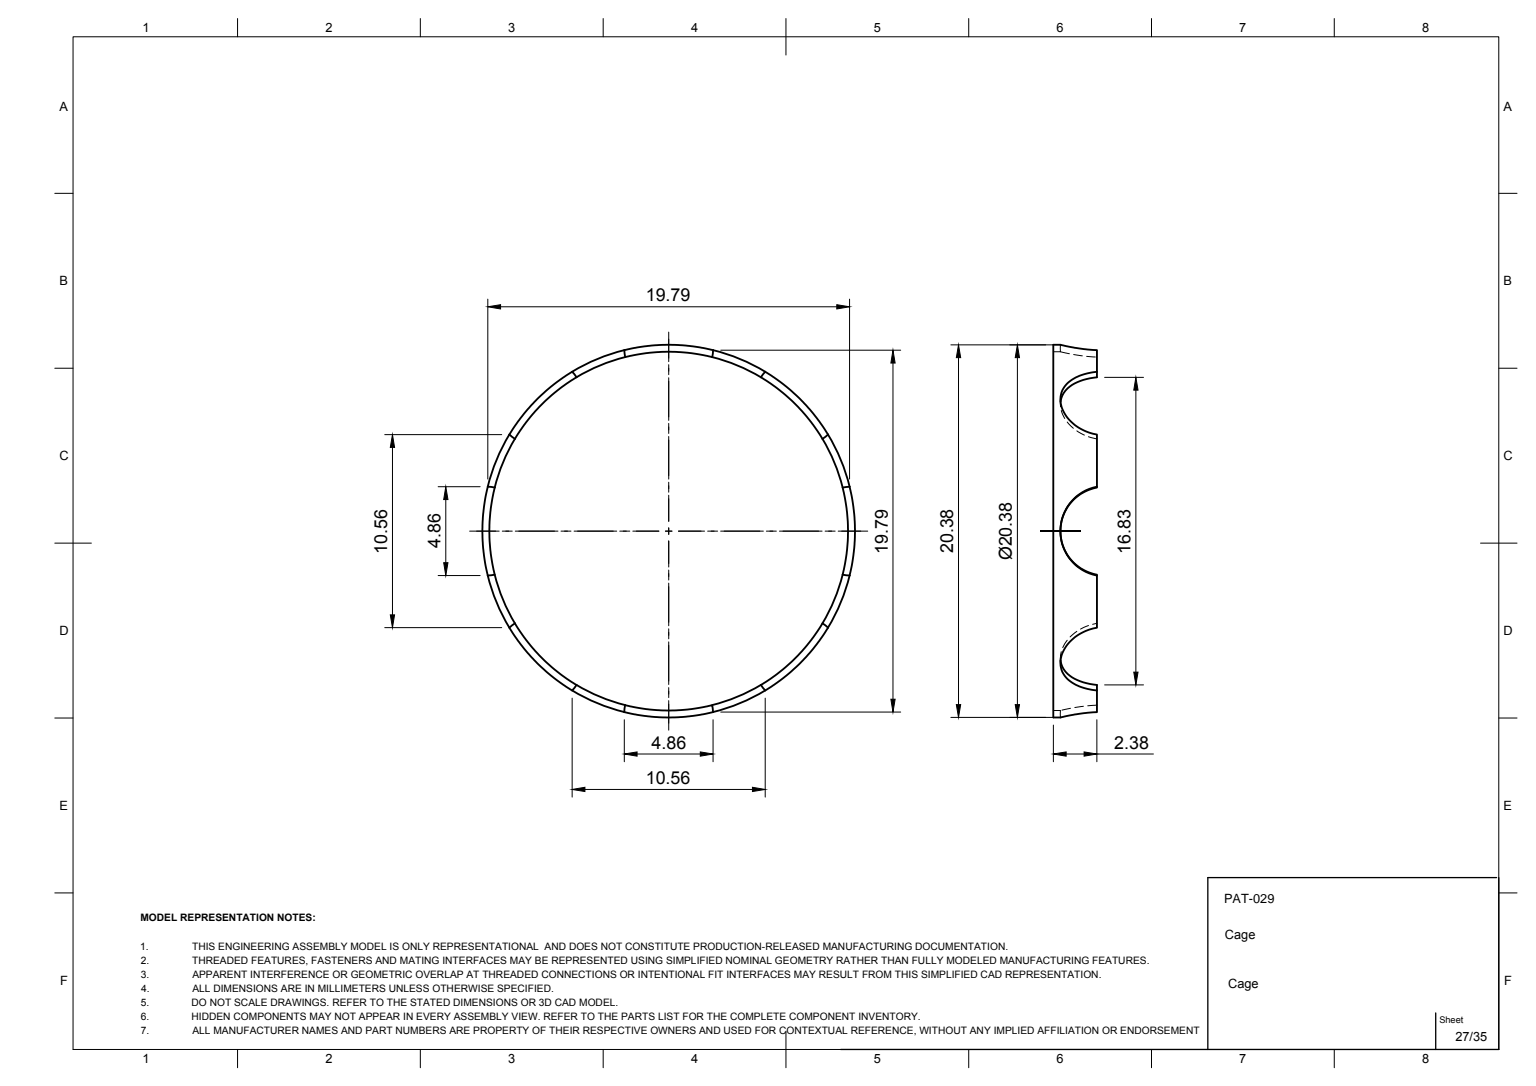
ISO-10303-21;
HEADER;
/* Generated by software containing ST-Developer
 * from STEP Tools, Inc. (www.steptools.com) 
 */

FILE_DESCRIPTION(
/* description */ ('Door-style hinge test fixture with detent'),
/* implementation_level */ '2;1');

FILE_NAME(
/* name */ 'Cage.step',
/* time_stamp */ '2026-10-28T03:24:57-07:00',
/* author */ (''),
/* organization */ (''),
/* preprocessor_version */ 'ST-DEVELOPER v20.2',
/* originating_system */ 'Autodesk Translation Framework v15.17.0.0',
/* authorisation */ '');

FILE_SCHEMA (('AUTOMOTIVE_DESIGN { 1 0 10303 214 3 1 1 }'));
ENDSEC;

DATA;
#10=MECHANICAL_DESIGN_GEOMETRIC_PRESENTATION_REPRESENTATION('',(#352),#9813);
#222=B_SPLINE_CURVE_WITH_KNOTS('',3,(#8878,#8879,#8880,#8881,#8882,#8883,
#8884,#8885,#8886,#8887,#8888,#8889,#8890,#8891,#8892,#8893,#8894,#8895,
#8896,#8897,#8898,#8899),.UNSPECIFIED.,.F.,.F.,(4,2,2,2,2,2,2,2,2,2,4),
(0.0473477652366656,0.126350602536658,0.189525903804987,0.252701205073317,
0.313298422430275,0.373895639787233,0.434492857144191,0.495090074501149,
0.558265375769478,0.621440677037807,0.7004435143378),.UNSPECIFIED.);
#223=B_SPLINE_CURVE_WITH_KNOTS('',3,(#8903,#8904,#8905,#8906,#8907,#8908,
#8909,#8910,#8911,#8912,#8913,#8914,#8915,#8916,#8917,#8918,#8919,#8920,
#8921,#8922,#8923,#8924),.UNSPECIFIED.,.F.,.F.,(4,2,2,2,2,2,2,2,2,2,4),
(0.0464897534940957,0.0852567806515119,0.170513561303024,0.246687263103517,
0.308657850341199,0.370628437578881,0.432599024816563,0.494569612054245,
0.570743313854739,0.656000094506251,0.694767121663666),.UNSPECIFIED.);
#224=B_SPLINE_CURVE_WITH_KNOTS('',3,(#8930,#8931,#8932,#8933,#8934,#8935,
#8936,#8937,#8938,#8939,#8940,#8941,#8942,#8943,#8944,#8945,#8946,#8947,
#8948,#8949,#8950,#8951),.UNSPECIFIED.,.F.,.F.,(4,2,2,2,2,2,2,2,2,2,4),
(0.0464897534940957,0.0852567806515118,0.170513561303024,0.246687263103517,
0.308657850341199,0.370628437578881,0.432599024816563,0.494569612054245,
0.570743313854738,0.65600009450625,0.694767121663666),.UNSPECIFIED.);
#225=B_SPLINE_CURVE_WITH_KNOTS('',3,(#8955,#8956,#8957,#8958,#8959,#8960,
#8961,#8962,#8963,#8964,#8965,#8966,#8967,#8968,#8969,#8970,#8971,#8972,
#8973,#8974,#8975,#8976),.UNSPECIFIED.,.F.,.F.,(4,2,2,2,2,2,2,2,2,2,4),
(0.0464897534940957,0.0852567806515119,0.170513561303024,0.246687263103517,
0.308657850341199,0.370628437578881,0.432599024816563,0.494569612054245,
0.570743313854739,0.656000094506251,0.694767121663666),.UNSPECIFIED.);
#226=B_SPLINE_CURVE_WITH_KNOTS('',3,(#8980,#8981,#8982,#8983,#8984,#8985,
#8986,#8987,#8988,#8989,#8990,#8991),.UNSPECIFIED.,.F.,.F.,(4,2,2,2,2,4),
(0.0464897534940957,0.0852567806515119,0.170513561303024,0.246687263103517,
0.308657850341199,0.370628437578881),.UNSPECIFIED.);
#227=B_SPLINE_CURVE_WITH_KNOTS('',3,(#8996,#8997,#8998,#8999,#9000,#9001,
#9002,#9003,#9004,#9005,#9006,#9007),.UNSPECIFIED.,.F.,.F.,(4,2,2,2,2,4),
(0.370628437578881,0.432599024816563,0.494569612054245,0.570743313854738,
0.65600009450625,0.694767121663666),.UNSPECIFIED.);
#228=B_SPLINE_CURVE_WITH_KNOTS('',3,(#9011,#9012,#9013,#9014,#9015,#9016,
#9017,#9018,#9019,#9020,#9021,#9022,#9023,#9024,#9025,#9026,#9027,#9028,
#9029,#9030,#9031,#9032),.UNSPECIFIED.,.F.,.F.,(4,2,2,2,2,2,2,2,2,2,4),
(0.0464897534940957,0.0852567806515121,0.170513561303024,0.246687263103518,
0.308657850341199,0.370628437578881,0.432599024816563,0.494569612054245,
0.570743313854738,0.65600009450625,0.694767121663666),.UNSPECIFIED.);
#229=B_SPLINE_CURVE_WITH_KNOTS('',3,(#9036,#9037,#9038,#9039,#9040,#9041,
#9042,#9043,#9044,#9045,#9046,#9047,#9048,#9049,#9050,#9051,#9052,#9053,
#9054,#9055,#9056,#9057),.UNSPECIFIED.,.F.,.F.,(4,2,2,2,2,2,2,2,2,2,4),
(0.0464897534940957,0.0852567806515119,0.170513561303024,0.246687263103517,
0.308657850341199,0.370628437578881,0.432599024816563,0.494569612054245,
0.570743313854738,0.65600009450625,0.694767121663667),.UNSPECIFIED.);
#230=B_SPLINE_CURVE_WITH_KNOTS('',3,(#9061,#9062,#9063,#9064,#9065,#9066,
#9067,#9068,#9069,#9070,#9071,#9072,#9073,#9074,#9075,#9076,#9077,#9078,
#9079,#9080,#9081,#9082),.UNSPECIFIED.,.F.,.F.,(4,2,2,2,2,2,2,2,2,2,4),
(0.0464897534940957,0.0852567806515119,0.170513561303024,0.246687263103517,
0.308657850341199,0.370628437578881,0.432599024816563,0.494569612054245,
0.570743313854738,0.65600009450625,0.694767121663666),.UNSPECIFIED.);
#231=B_SPLINE_CURVE_WITH_KNOTS('',3,(#9086,#9087,#9088,#9089,#9090,#9091,
#9092,#9093,#9094,#9095,#9096,#9097,#9098,#9099,#9100,#9101,#9102,#9103,
#9104,#9105,#9106,#9107),.UNSPECIFIED.,.F.,.F.,(4,2,2,2,2,2,2,2,2,2,4),
(0.0464897534940957,0.0852567806515119,0.170513561303024,0.246687263103517,
0.308657850341199,0.370628437578881,0.432599024816563,0.494569612054245,
0.570743313854739,0.656000094506251,0.694767121663667),.UNSPECIFIED.);
#232=B_SPLINE_CURVE_WITH_KNOTS('',3,(#9115,#9116,#9117,#9118,#9119,#9120,
#9121,#9122,#9123,#9124,#9125,#9126,#9127,#9128,#9129,#9130,#9131,#9132,
#9133,#9134,#9135,#9136),.UNSPECIFIED.,.F.,.F.,(4,2,2,2,2,2,2,2,2,2,4),
(0.0473477652366656,0.126350602536658,0.189525903804987,0.252701205073316,
0.313298422430274,0.373895639787232,0.434492857144191,0.495090074501149,
0.558265375769478,0.621440677037807,0.7004435143378),.UNSPECIFIED.);
#233=B_SPLINE_CURVE_WITH_KNOTS('',3,(#9144,#9145,#9146,#9147,#9148,#9149,
#9150,#9151,#9152,#9153,#9154,#9155,#9156,#9157,#9158,#9159,#9160,#9161,
#9162,#9163,#9164,#9165),.UNSPECIFIED.,.F.,.F.,(4,2,2,2,2,2,2,2,2,2,4),
(0.0473477652366656,0.126350602536658,0.189525903804987,0.252701205073317,
0.313298422430275,0.373895639787233,0.434492857144191,0.495090074501149,
0.558265375769478,0.621440677037807,0.7004435143378),.UNSPECIFIED.);
#234=B_SPLINE_CURVE_WITH_KNOTS('',3,(#9174,#9175,#9176,#9177,#9178,#9179,
#9180,#9181,#9182,#9183,#9184,#9185),.UNSPECIFIED.,.F.,.F.,(4,2,2,2,2,4),
(0.0473477652366656,0.126350602536658,0.189525903804987,0.252701205073316,
0.313298422430275,0.373895639787233),.UNSPECIFIED.);
#235=B_SPLINE_CURVE_WITH_KNOTS('',3,(#9187,#9188,#9189,#9190,#9191,#9192,
#9193,#9194,#9195,#9196,#9197,#9198),.UNSPECIFIED.,.F.,.F.,(4,2,2,2,2,4),
(0.373895639787233,0.434492857144191,0.495090074501149,0.558265375769478,
0.621440677037807,0.7004435143378),.UNSPECIFIED.);
#236=B_SPLINE_CURVE_WITH_KNOTS('',3,(#9205,#9206,#9207,#9208,#9209,#9210,
#9211,#9212,#9213,#9214,#9215,#9216,#9217,#9218,#9219,#9220,#9221,#9222,
#9223,#9224,#9225,#9226),.UNSPECIFIED.,.F.,.F.,(4,2,2,2,2,2,2,2,2,2,4),
(0.0473477652366656,0.126350602536658,0.189525903804987,0.252701205073316,
0.313298422430275,0.373895639787233,0.434492857144191,0.495090074501149,
0.558265375769478,0.621440677037807,0.7004435143378),.UNSPECIFIED.);
#237=B_SPLINE_CURVE_WITH_KNOTS('',3,(#9234,#9235,#9236,#9237,#9238,#9239,
#9240,#9241,#9242,#9243,#9244,#9245,#9246,#9247,#9248,#9249,#9250,#9251,
#9252,#9253,#9254,#9255),.UNSPECIFIED.,.F.,.F.,(4,2,2,2,2,2,2,2,2,2,4),
(0.0473477652366656,0.126350602536658,0.189525903804987,0.252701205073317,
0.313298422430275,0.373895639787233,0.434492857144191,0.495090074501149,
0.558265375769478,0.621440677037807,0.7004435143378),.UNSPECIFIED.);
#238=B_SPLINE_CURVE_WITH_KNOTS('',3,(#9263,#9264,#9265,#9266,#9267,#9268,
#9269,#9270,#9271,#9272,#9273,#9274,#9275,#9276,#9277,#9278,#9279,#9280,
#9281,#9282,#9283,#9284),.UNSPECIFIED.,.F.,.F.,(4,2,2,2,2,2,2,2,2,2,4),
(0.0473477652366656,0.126350602536658,0.189525903804987,0.252701205073316,
0.313298422430275,0.373895639787233,0.434492857144191,0.495090074501149,
0.558265375769478,0.621440677037807,0.7004435143378),.UNSPECIFIED.);
#239=B_SPLINE_CURVE_WITH_KNOTS('',3,(#9293,#9294,#9295,#9296,#9297,#9298,
#9299,#9300,#9301,#9302,#9303,#9304,#9305,#9306,#9307,#9308,#9309,#9310,
#9311,#9312,#9313,#9314),.UNSPECIFIED.,.F.,.F.,(4,2,2,2,2,2,2,2,2,2,4),
(0.0473477652366656,0.126350602536658,0.189525903804987,0.252701205073317,
0.313298422430275,0.373895639787233,0.434492857144191,0.495090074501149,
0.558265375769478,0.621440677037807,0.7004435143378),.UNSPECIFIED.);
#251=SPHERICAL_SURFACE('',#5501,0.247676);
#252=SPHERICAL_SURFACE('',#5517,0.247676);
#253=SPHERICAL_SURFACE('',#5522,0.247676);
#254=SPHERICAL_SURFACE('',#5527,0.247676);
#255=SPHERICAL_SURFACE('',#5532,0.247676);
#256=SPHERICAL_SURFACE('',#5537,0.247676);
#257=SPHERICAL_SURFACE('',#5542,0.247676);
#258=SPHERICAL_SURFACE('',#5550,0.247676);
#282=SHAPE_REPRESENTATION_RELATIONSHIP('SRR','None',#9960,#313);
#313=ADVANCED_BREP_SHAPE_REPRESENTATION('',(#391),#9803);
#352=STYLED_ITEM('',(#10183),#391);
#391=MANIFOLD_SOLID_BREP('Continuous crown cage',#4784);
#472=FACE_BOUND('',#1225,.T.);
#609=PLANE('',#5514);
#610=PLANE('',#5519);
#611=PLANE('',#5524);
#612=PLANE('',#5529);
#613=PLANE('',#5534);
#614=PLANE('',#5539);
#615=PLANE('',#5548);
#616=PLANE('',#5552);
#617=PLANE('',#5553);
#849=FACE_OUTER_BOUND('',#1207,.T.);
#850=FACE_OUTER_BOUND('',#1208,.T.);
#851=FACE_OUTER_BOUND('',#1209,.T.);
#852=FACE_OUTER_BOUND('',#1210,.T.);
#853=FACE_OUTER_BOUND('',#1211,.T.);
#854=FACE_OUTER_BOUND('',#1212,.T.);
#855=FACE_OUTER_BOUND('',#1213,.T.);
#856=FACE_OUTER_BOUND('',#1214,.T.);
#857=FACE_OUTER_BOUND('',#1215,.T.);
#858=FACE_OUTER_BOUND('',#1216,.T.);
#859=FACE_OUTER_BOUND('',#1217,.T.);
#860=FACE_OUTER_BOUND('',#1218,.T.);
#861=FACE_OUTER_BOUND('',#1219,.T.);
#862=FACE_OUTER_BOUND('',#1220,.T.);
#863=FACE_OUTER_BOUND('',#1221,.T.);
#864=FACE_OUTER_BOUND('',#1222,.T.);
#865=FACE_OUTER_BOUND('',#1223,.T.);
#866=FACE_OUTER_BOUND('',#1224,.T.);
#867=FACE_OUTER_BOUND('',#1226,.T.);
#1207=EDGE_LOOP('',(#3979,#3980,#3981,#3982));
#1208=EDGE_LOOP('',(#3983,#3984,#3985,#3986,#3987,#3988,#3989,#3990,#3991,
#3992,#3993,#3994,#3995,#3996,#3997,#3998,#3999,#4000,#4001,#4002));
#1209=EDGE_LOOP('',(#4003,#4004,#4005,#4006));
#1210=EDGE_LOOP('',(#4007,#4008,#4009,#4010));
#1211=EDGE_LOOP('',(#4011,#4012,#4013,#4014));
#1212=EDGE_LOOP('',(#4015,#4016,#4017,#4018));
#1213=EDGE_LOOP('',(#4019,#4020,#4021,#4022));
#1214=EDGE_LOOP('',(#4023,#4024,#4025,#4026,#4027,#4028));
#1215=EDGE_LOOP('',(#4029,#4030,#4031,#4032));
#1216=EDGE_LOOP('',(#4033,#4034,#4035,#4036));
#1217=EDGE_LOOP('',(#4037,#4038,#4039,#4040));
#1218=EDGE_LOOP('',(#4041,#4042,#4043,#4044));
#1219=EDGE_LOOP('',(#4045,#4046,#4047,#4048));
#1220=EDGE_LOOP('',(#4049,#4050,#4051,#4052));
#1221=EDGE_LOOP('',(#4053,#4054,#4055,#4056,#4057,#4058,#4059,#4060,#4061,
#4062,#4063,#4064,#4065,#4066,#4067,#4068,#4069,#4070,#4071,#4072));
#1222=EDGE_LOOP('',(#4073,#4074,#4075,#4076));
#1223=EDGE_LOOP('',(#4077,#4078,#4079,#4080));
#1224=EDGE_LOOP('',(#4081));
#1225=EDGE_LOOP('',(#4082));
#1226=EDGE_LOOP('',(#4083,#4084,#4085,#4086));
#1567=LINE('',#8993,#1887);
#1568=LINE('',#9289,#1888);
#1887=VECTOR('',#6724,1.019052);
#1888=VECTOR('',#6801,0.980948);
#2126=CIRCLE('',#5502,0.243053047864041);
#2127=CIRCLE('',#5503,0.243053047864041);
#2128=CIRCLE('',#5505,1.019052);
#2129=CIRCLE('',#5506,1.019052);
#2130=CIRCLE('',#5507,1.019052);
#2131=CIRCLE('',#5508,1.019052);
#2132=CIRCLE('',#5509,1.019052);
#2133=CIRCLE('',#5510,1.019052);
#2134=CIRCLE('',#5511,1.019052);
#2135=CIRCLE('',#5512,1.019052);
#2136=CIRCLE('',#5513,1.019052);
#2137=CIRCLE('',#5515,0.980948);
#2138=CIRCLE('',#5516,0.243053047864041);
#2139=CIRCLE('',#5518,0.243053047864041);
#2140=CIRCLE('',#5520,0.980948);
#2141=CIRCLE('',#5521,0.243053047864041);
#2142=CIRCLE('',#5523,0.243053047864041);
#2143=CIRCLE('',#5525,0.980948);
#2144=CIRCLE('',#5526,0.243053047864041);
#2145=CIRCLE('',#5528,0.243053047864041);
#2146=CIRCLE('',#5530,0.980948);
#2147=CIRCLE('',#5531,0.243053047864041);
#2148=CIRCLE('',#5533,0.243053047864041);
#2149=CIRCLE('',#5535,0.980948);
#2150=CIRCLE('',#5536,0.243053047864041);
#2151=CIRCLE('',#5538,0.243053047864041);
#2152=CIRCLE('',#5540,0.980948);
#2153=CIRCLE('',#5541,0.243053047864041);
#2154=CIRCLE('',#5543,0.243053047864041);
#2155=CIRCLE('',#5545,0.980948);
#2156=CIRCLE('',#5546,0.980948);
#2157=CIRCLE('',#5547,0.980948);
#2158=CIRCLE('',#5549,0.243053047864041);
#2159=CIRCLE('',#5551,0.243053047864041);
#2488=VERTEX_POINT('',#8876);
#2489=VERTEX_POINT('',#8877);
#2490=VERTEX_POINT('',#8900);
#2491=VERTEX_POINT('',#8902);
#2492=VERTEX_POINT('',#8927);
#2493=VERTEX_POINT('',#8929);
#2494=VERTEX_POINT('',#8952);
#2495=VERTEX_POINT('',#8954);
#2496=VERTEX_POINT('',#8977);
#2497=VERTEX_POINT('',#8979);
#2498=VERTEX_POINT('',#8992);
#2499=VERTEX_POINT('',#8995);
#2500=VERTEX_POINT('',#9008);
#2501=VERTEX_POINT('',#9010);
#2502=VERTEX_POINT('',#9033);
#2503=VERTEX_POINT('',#9035);
#2504=VERTEX_POINT('',#9058);
#2505=VERTEX_POINT('',#9060);
#2506=VERTEX_POINT('',#9083);
#2507=VERTEX_POINT('',#9085);
#2508=VERTEX_POINT('',#9110);
#2509=VERTEX_POINT('',#9114);
#2510=VERTEX_POINT('',#9139);
#2511=VERTEX_POINT('',#9143);
#2512=VERTEX_POINT('',#9168);
#2513=VERTEX_POINT('',#9172);
#2514=VERTEX_POINT('',#9173);
#2515=VERTEX_POINT('',#9200);
#2516=VERTEX_POINT('',#9204);
#2517=VERTEX_POINT('',#9229);
#2518=VERTEX_POINT('',#9233);
#2519=VERTEX_POINT('',#9258);
#2520=VERTEX_POINT('',#9262);
#2521=VERTEX_POINT('',#9287);
#2522=VERTEX_POINT('',#9290);
#2523=VERTEX_POINT('',#9292);
#3006=EDGE_CURVE('',#2488,#2489,#222,.T.);
#3007=EDGE_CURVE('',#2490,#2488,#2126,.T.);
#3008=EDGE_CURVE('',#2491,#2490,#223,.T.);
#3009=EDGE_CURVE('',#2489,#2491,#2127,.T.);
#3010=EDGE_CURVE('',#2492,#2490,#2128,.T.);
#3011=EDGE_CURVE('',#2492,#2493,#224,.T.);
#3012=EDGE_CURVE('',#2494,#2493,#2129,.T.);
#3013=EDGE_CURVE('',#2494,#2495,#225,.T.);
#3014=EDGE_CURVE('',#2496,#2495,#2130,.T.);
#3015=EDGE_CURVE('',#2496,#2497,#226,.T.);
#3016=EDGE_CURVE('',#2497,#2498,#1567,.T.);
#3017=EDGE_CURVE('',#2498,#2498,#2131,.T.);
#3018=EDGE_CURVE('',#2497,#2499,#227,.T.);
#3019=EDGE_CURVE('',#2500,#2499,#2132,.T.);
#3020=EDGE_CURVE('',#2500,#2501,#228,.T.);
#3021=EDGE_CURVE('',#2502,#2501,#2133,.T.);
#3022=EDGE_CURVE('',#2502,#2503,#229,.T.);
#3023=EDGE_CURVE('',#2504,#2503,#2134,.T.);
#3024=EDGE_CURVE('',#2504,#2505,#230,.T.);
#3025=EDGE_CURVE('',#2506,#2505,#2135,.T.);
#3026=EDGE_CURVE('',#2506,#2507,#231,.T.);
#3027=EDGE_CURVE('',#2491,#2507,#2136,.T.);
#3028=EDGE_CURVE('',#2488,#2508,#2137,.T.);
#3029=EDGE_CURVE('',#2508,#2492,#2138,.T.);
#3030=EDGE_CURVE('',#2509,#2508,#232,.T.);
#3031=EDGE_CURVE('',#2493,#2509,#2139,.T.);
#3032=EDGE_CURVE('',#2509,#2510,#2140,.T.);
#3033=EDGE_CURVE('',#2510,#2494,#2141,.T.);
#3034=EDGE_CURVE('',#2511,#2510,#233,.T.);
#3035=EDGE_CURVE('',#2495,#2511,#2142,.T.);
#3036=EDGE_CURVE('',#2511,#2512,#2143,.T.);
#3037=EDGE_CURVE('',#2512,#2496,#2144,.T.);
#3038=EDGE_CURVE('',#2513,#2514,#234,.T.);
#3039=EDGE_CURVE('',#2499,#2513,#2145,.T.);
#3040=EDGE_CURVE('',#2514,#2512,#235,.T.);
#3041=EDGE_CURVE('',#2513,#2515,#2146,.T.);
#3042=EDGE_CURVE('',#2515,#2500,#2147,.T.);
#3043=EDGE_CURVE('',#2516,#2515,#236,.T.);
#3044=EDGE_CURVE('',#2501,#2516,#2148,.T.);
#3045=EDGE_CURVE('',#2516,#2517,#2149,.T.);
#3046=EDGE_CURVE('',#2517,#2502,#2150,.T.);
#3047=EDGE_CURVE('',#2518,#2517,#237,.T.);
#3048=EDGE_CURVE('',#2503,#2518,#2151,.T.);
#3049=EDGE_CURVE('',#2518,#2519,#2152,.T.);
#3050=EDGE_CURVE('',#2519,#2504,#2153,.T.);
#3051=EDGE_CURVE('',#2520,#2519,#238,.T.);
#3052=EDGE_CURVE('',#2505,#2520,#2154,.T.);
#3053=EDGE_CURVE('',#2521,#2521,#2155,.T.);
#3054=EDGE_CURVE('',#2521,#2514,#1568,.T.);
#3055=EDGE_CURVE('',#2522,#2489,#2156,.T.);
#3056=EDGE_CURVE('',#2522,#2523,#239,.T.);
#3057=EDGE_CURVE('',#2520,#2523,#2157,.T.);
#3058=EDGE_CURVE('',#2507,#2522,#2158,.T.);
#3059=EDGE_CURVE('',#2523,#2506,#2159,.T.);
#3979=ORIENTED_EDGE('',*,*,#3006,.F.);
#3980=ORIENTED_EDGE('',*,*,#3007,.F.);
#3981=ORIENTED_EDGE('',*,*,#3008,.F.);
#3982=ORIENTED_EDGE('',*,*,#3009,.F.);
#3983=ORIENTED_EDGE('',*,*,#3008,.T.);
#3984=ORIENTED_EDGE('',*,*,#3010,.F.);
#3985=ORIENTED_EDGE('',*,*,#3011,.T.);
#3986=ORIENTED_EDGE('',*,*,#3012,.F.);
#3987=ORIENTED_EDGE('',*,*,#3013,.T.);
#3988=ORIENTED_EDGE('',*,*,#3014,.F.);
#3989=ORIENTED_EDGE('',*,*,#3015,.T.);
#3990=ORIENTED_EDGE('',*,*,#3016,.T.);
#3991=ORIENTED_EDGE('',*,*,#3017,.F.);
#3992=ORIENTED_EDGE('',*,*,#3016,.F.);
#3993=ORIENTED_EDGE('',*,*,#3018,.T.);
#3994=ORIENTED_EDGE('',*,*,#3019,.F.);
#3995=ORIENTED_EDGE('',*,*,#3020,.T.);
#3996=ORIENTED_EDGE('',*,*,#3021,.F.);
#3997=ORIENTED_EDGE('',*,*,#3022,.T.);
#3998=ORIENTED_EDGE('',*,*,#3023,.F.);
#3999=ORIENTED_EDGE('',*,*,#3024,.T.);
#4000=ORIENTED_EDGE('',*,*,#3025,.F.);
#4001=ORIENTED_EDGE('',*,*,#3026,.T.);
#4002=ORIENTED_EDGE('',*,*,#3027,.F.);
#4003=ORIENTED_EDGE('',*,*,#3007,.T.);
#4004=ORIENTED_EDGE('',*,*,#3028,.T.);
#4005=ORIENTED_EDGE('',*,*,#3029,.T.);
#4006=ORIENTED_EDGE('',*,*,#3010,.T.);
#4007=ORIENTED_EDGE('',*,*,#3030,.F.);
#4008=ORIENTED_EDGE('',*,*,#3031,.F.);
#4009=ORIENTED_EDGE('',*,*,#3011,.F.);
#4010=ORIENTED_EDGE('',*,*,#3029,.F.);
#4011=ORIENTED_EDGE('',*,*,#3031,.T.);
#4012=ORIENTED_EDGE('',*,*,#3032,.T.);
#4013=ORIENTED_EDGE('',*,*,#3033,.T.);
#4014=ORIENTED_EDGE('',*,*,#3012,.T.);
#4015=ORIENTED_EDGE('',*,*,#3034,.F.);
#4016=ORIENTED_EDGE('',*,*,#3035,.F.);
#4017=ORIENTED_EDGE('',*,*,#3013,.F.);
#4018=ORIENTED_EDGE('',*,*,#3033,.F.);
#4019=ORIENTED_EDGE('',*,*,#3035,.T.);
#4020=ORIENTED_EDGE('',*,*,#3036,.T.);
#4021=ORIENTED_EDGE('',*,*,#3037,.T.);
#4022=ORIENTED_EDGE('',*,*,#3014,.T.);
#4023=ORIENTED_EDGE('',*,*,#3038,.F.);
#4024=ORIENTED_EDGE('',*,*,#3039,.F.);
#4025=ORIENTED_EDGE('',*,*,#3018,.F.);
#4026=ORIENTED_EDGE('',*,*,#3015,.F.);
#4027=ORIENTED_EDGE('',*,*,#3037,.F.);
#4028=ORIENTED_EDGE('',*,*,#3040,.F.);
#4029=ORIENTED_EDGE('',*,*,#3039,.T.);
#4030=ORIENTED_EDGE('',*,*,#3041,.T.);
#4031=ORIENTED_EDGE('',*,*,#3042,.T.);
#4032=ORIENTED_EDGE('',*,*,#3019,.T.);
#4033=ORIENTED_EDGE('',*,*,#3043,.F.);
#4034=ORIENTED_EDGE('',*,*,#3044,.F.);
#4035=ORIENTED_EDGE('',*,*,#3020,.F.);
#4036=ORIENTED_EDGE('',*,*,#3042,.F.);
#4037=ORIENTED_EDGE('',*,*,#3044,.T.);
#4038=ORIENTED_EDGE('',*,*,#3045,.T.);
#4039=ORIENTED_EDGE('',*,*,#3046,.T.);
#4040=ORIENTED_EDGE('',*,*,#3021,.T.);
#4041=ORIENTED_EDGE('',*,*,#3047,.F.);
#4042=ORIENTED_EDGE('',*,*,#3048,.F.);
#4043=ORIENTED_EDGE('',*,*,#3022,.F.);
#4044=ORIENTED_EDGE('',*,*,#3046,.F.);
#4045=ORIENTED_EDGE('',*,*,#3048,.T.);
#4046=ORIENTED_EDGE('',*,*,#3049,.T.);
#4047=ORIENTED_EDGE('',*,*,#3050,.T.);
#4048=ORIENTED_EDGE('',*,*,#3023,.T.);
#4049=ORIENTED_EDGE('',*,*,#3024,.F.);
#4050=ORIENTED_EDGE('',*,*,#3050,.F.);
#4051=ORIENTED_EDGE('',*,*,#3051,.F.);
#4052=ORIENTED_EDGE('',*,*,#3052,.F.);
#4053=ORIENTED_EDGE('',*,*,#3053,.F.);
#4054=ORIENTED_EDGE('',*,*,#3054,.T.);
#4055=ORIENTED_EDGE('',*,*,#3040,.T.);
#4056=ORIENTED_EDGE('',*,*,#3036,.F.);
#4057=ORIENTED_EDGE('',*,*,#3034,.T.);
#4058=ORIENTED_EDGE('',*,*,#3032,.F.);
#4059=ORIENTED_EDGE('',*,*,#3030,.T.);
#4060=ORIENTED_EDGE('',*,*,#3028,.F.);
#4061=ORIENTED_EDGE('',*,*,#3006,.T.);
#4062=ORIENTED_EDGE('',*,*,#3055,.F.);
#4063=ORIENTED_EDGE('',*,*,#3056,.T.);
#4064=ORIENTED_EDGE('',*,*,#3057,.F.);
#4065=ORIENTED_EDGE('',*,*,#3051,.T.);
#4066=ORIENTED_EDGE('',*,*,#3049,.F.);
#4067=ORIENTED_EDGE('',*,*,#3047,.T.);
#4068=ORIENTED_EDGE('',*,*,#3045,.F.);
#4069=ORIENTED_EDGE('',*,*,#3043,.T.);
#4070=ORIENTED_EDGE('',*,*,#3041,.F.);
#4071=ORIENTED_EDGE('',*,*,#3038,.T.);
#4072=ORIENTED_EDGE('',*,*,#3054,.F.);
#4073=ORIENTED_EDGE('',*,*,#3009,.T.);
#4074=ORIENTED_EDGE('',*,*,#3027,.T.);
#4075=ORIENTED_EDGE('',*,*,#3058,.T.);
#4076=ORIENTED_EDGE('',*,*,#3055,.T.);
#4077=ORIENTED_EDGE('',*,*,#3026,.F.);
#4078=ORIENTED_EDGE('',*,*,#3059,.F.);
#4079=ORIENTED_EDGE('',*,*,#3056,.F.);
#4080=ORIENTED_EDGE('',*,*,#3058,.F.);
#4081=ORIENTED_EDGE('',*,*,#3017,.T.);
#4082=ORIENTED_EDGE('',*,*,#3053,.T.);
#4083=ORIENTED_EDGE('',*,*,#3052,.T.);
#4084=ORIENTED_EDGE('',*,*,#3057,.T.);
#4085=ORIENTED_EDGE('',*,*,#3059,.T.);
#4086=ORIENTED_EDGE('',*,*,#3025,.T.);
#4439=CYLINDRICAL_SURFACE('',#5504,1.019052);
#4440=CYLINDRICAL_SURFACE('',#5544,0.980948);
#4654=ADVANCED_FACE('',(#849),#251,.F.);
#4655=ADVANCED_FACE('',(#850),#4439,.T.);
#4656=ADVANCED_FACE('',(#851),#609,.T.);
#4657=ADVANCED_FACE('',(#852),#252,.F.);
#4658=ADVANCED_FACE('',(#853),#610,.T.);
#4659=ADVANCED_FACE('',(#854),#253,.F.);
#4660=ADVANCED_FACE('',(#855),#611,.T.);
#4661=ADVANCED_FACE('',(#856),#254,.F.);
#4662=ADVANCED_FACE('',(#857),#612,.T.);
#4663=ADVANCED_FACE('',(#858),#255,.F.);
#4664=ADVANCED_FACE('',(#859),#613,.T.);
#4665=ADVANCED_FACE('',(#860),#256,.F.);
#4666=ADVANCED_FACE('',(#861),#614,.T.);
#4667=ADVANCED_FACE('',(#862),#257,.F.);
#4668=ADVANCED_FACE('',(#863),#4440,.F.);
#4669=ADVANCED_FACE('',(#864),#615,.T.);
#4670=ADVANCED_FACE('',(#865),#258,.F.);
#4671=ADVANCED_FACE('',(#866,#472),#616,.T.);
#4672=ADVANCED_FACE('',(#867),#617,.T.);
#4784=CLOSED_SHELL('',(#4654,#4655,#4656,#4657,#4658,#4659,#4660,#4661,
#4662,#4663,#4664,#4665,#4666,#4667,#4668,#4669,#4670,#4671,#4672));
#5500=AXIS2_PLACEMENT_3D('',#8874,#6708,#6709);
#5501=AXIS2_PLACEMENT_3D('',#8875,#6710,#6711);
#5502=AXIS2_PLACEMENT_3D('',#8901,#6712,#6713);
#5503=AXIS2_PLACEMENT_3D('',#8925,#6714,#6715);
#5504=AXIS2_PLACEMENT_3D('',#8926,#6716,#6717);
#5505=AXIS2_PLACEMENT_3D('',#8928,#6718,#6719);
#5506=AXIS2_PLACEMENT_3D('',#8953,#6720,#6721);
#5507=AXIS2_PLACEMENT_3D('',#8978,#6722,#6723);
#5508=AXIS2_PLACEMENT_3D('',#8994,#6725,#6726);
#5509=AXIS2_PLACEMENT_3D('',#9009,#6727,#6728);
#5510=AXIS2_PLACEMENT_3D('',#9034,#6729,#6730);
#5511=AXIS2_PLACEMENT_3D('',#9059,#6731,#6732);
#5512=AXIS2_PLACEMENT_3D('',#9084,#6733,#6734);
#5513=AXIS2_PLACEMENT_3D('',#9108,#6735,#6736);
#5514=AXIS2_PLACEMENT_3D('',#9109,#6737,#6738);
#5515=AXIS2_PLACEMENT_3D('',#9111,#6739,#6740);
#5516=AXIS2_PLACEMENT_3D('',#9112,#6741,#6742);
#5517=AXIS2_PLACEMENT_3D('',#9113,#6743,#6744);
#5518=AXIS2_PLACEMENT_3D('',#9137,#6745,#6746);
#5519=AXIS2_PLACEMENT_3D('',#9138,#6747,#6748);
#5520=AXIS2_PLACEMENT_3D('',#9140,#6749,#6750);
#5521=AXIS2_PLACEMENT_3D('',#9141,#6751,#6752);
#5522=AXIS2_PLACEMENT_3D('',#9142,#6753,#6754);
#5523=AXIS2_PLACEMENT_3D('',#9166,#6755,#6756);
#5524=AXIS2_PLACEMENT_3D('',#9167,#6757,#6758);
#5525=AXIS2_PLACEMENT_3D('',#9169,#6759,#6760);
#5526=AXIS2_PLACEMENT_3D('',#9170,#6761,#6762);
#5527=AXIS2_PLACEMENT_3D('',#9171,#6763,#6764);
#5528=AXIS2_PLACEMENT_3D('',#9186,#6765,#6766);
#5529=AXIS2_PLACEMENT_3D('',#9199,#6767,#6768);
#5530=AXIS2_PLACEMENT_3D('',#9201,#6769,#6770);
#5531=AXIS2_PLACEMENT_3D('',#9202,#6771,#6772);
#5532=AXIS2_PLACEMENT_3D('',#9203,#6773,#6774);
#5533=AXIS2_PLACEMENT_3D('',#9227,#6775,#6776);
#5534=AXIS2_PLACEMENT_3D('',#9228,#6777,#6778);
#5535=AXIS2_PLACEMENT_3D('',#9230,#6779,#6780);
#5536=AXIS2_PLACEMENT_3D('',#9231,#6781,#6782);
#5537=AXIS2_PLACEMENT_3D('',#9232,#6783,#6784);
#5538=AXIS2_PLACEMENT_3D('',#9256,#6785,#6786);
#5539=AXIS2_PLACEMENT_3D('',#9257,#6787,#6788);
#5540=AXIS2_PLACEMENT_3D('',#9259,#6789,#6790);
#5541=AXIS2_PLACEMENT_3D('',#9260,#6791,#6792);
#5542=AXIS2_PLACEMENT_3D('',#9261,#6793,#6794);
#5543=AXIS2_PLACEMENT_3D('',#9285,#6795,#6796);
#5544=AXIS2_PLACEMENT_3D('',#9286,#6797,#6798);
#5545=AXIS2_PLACEMENT_3D('',#9288,#6799,#6800);
#5546=AXIS2_PLACEMENT_3D('',#9291,#6802,#6803);
#5547=AXIS2_PLACEMENT_3D('',#9315,#6804,#6805);
#5548=AXIS2_PLACEMENT_3D('',#9316,#6806,#6807);
#5549=AXIS2_PLACEMENT_3D('',#9317,#6808,#6809);
#5550=AXIS2_PLACEMENT_3D('',#9318,#6810,#6811);
#5551=AXIS2_PLACEMENT_3D('',#9319,#6812,#6813);
#5552=AXIS2_PLACEMENT_3D('',#9320,#6814,#6815);
#5553=AXIS2_PLACEMENT_3D('',#9321,#6816,#6817);
#6708=DIRECTION('axis',(0.,0.,1.));
#6709=DIRECTION('refdir',(1.,0.,0.));
#6710=DIRECTION('center_axis',(0.,0.,1.));
#6711=DIRECTION('ref_axis',(1.,0.,0.));
#6712=DIRECTION('center_axis',(0.,-1.,0.));
#6713=DIRECTION('ref_axis',(0.,0.,-1.));
#6714=DIRECTION('center_axis',(0.,-1.,0.));
#6715=DIRECTION('ref_axis',(0.,0.,-1.));
#6716=DIRECTION('center_axis',(0.,1.,0.));
#6717=DIRECTION('ref_axis',(1.,0.,0.));
#6718=DIRECTION('center_axis',(0.,1.,0.));
#6719=DIRECTION('ref_axis',(1.,0.,0.));
#6720=DIRECTION('center_axis',(0.,1.,0.));
#6721=DIRECTION('ref_axis',(1.,0.,0.));
#6722=DIRECTION('center_axis',(0.,1.,0.));
#6723=DIRECTION('ref_axis',(1.,0.,0.));
#6724=DIRECTION('',(0.,-1.,0.));
#6725=DIRECTION('center_axis',(0.,-1.,0.));
#6726=DIRECTION('ref_axis',(1.,0.,0.));
#6727=DIRECTION('center_axis',(0.,1.,0.));
#6728=DIRECTION('ref_axis',(1.,0.,0.));
#6729=DIRECTION('center_axis',(0.,1.,0.));
#6730=DIRECTION('ref_axis',(1.,0.,0.));
#6731=DIRECTION('center_axis',(0.,1.,0.));
#6732=DIRECTION('ref_axis',(1.,0.,0.));
#6733=DIRECTION('center_axis',(0.,1.,0.));
#6734=DIRECTION('ref_axis',(1.,0.,0.));
#6735=DIRECTION('center_axis',(0.,1.,0.));
#6736=DIRECTION('ref_axis',(1.,0.,0.));
#6737=DIRECTION('center_axis',(0.,1.,0.));
#6738=DIRECTION('ref_axis',(1.,0.,0.));
#6739=DIRECTION('center_axis',(0.,-1.,0.));
#6740=DIRECTION('ref_axis',(1.,0.,0.));
#6741=DIRECTION('center_axis',(0.,-1.,0.));
#6742=DIRECTION('ref_axis',(0.,0.,-1.));
#6743=DIRECTION('center_axis',(6.12323399573677E-17,0.,1.));
#6744=DIRECTION('ref_axis',(1.,0.,0.));
#6745=DIRECTION('center_axis',(0.,-1.,0.));
#6746=DIRECTION('ref_axis',(0.,0.,-1.));
#6747=DIRECTION('center_axis',(0.,1.,0.));
#6748=DIRECTION('ref_axis',(1.,0.,0.));
#6749=DIRECTION('center_axis',(0.,-1.,0.));
#6750=DIRECTION('ref_axis',(1.,0.,0.));
#6751=DIRECTION('center_axis',(0.,-1.,0.));
#6752=DIRECTION('ref_axis',(0.,0.,-1.));
#6753=DIRECTION('center_axis',(0.,0.,1.));
#6754=DIRECTION('ref_axis',(1.,0.,0.));
#6755=DIRECTION('center_axis',(0.,-1.,0.));
#6756=DIRECTION('ref_axis',(0.,0.,-1.));
#6757=DIRECTION('center_axis',(0.,1.,0.));
#6758=DIRECTION('ref_axis',(1.,0.,0.));
#6759=DIRECTION('center_axis',(0.,-1.,0.));
#6760=DIRECTION('ref_axis',(1.,0.,0.));
#6761=DIRECTION('center_axis',(0.,-1.,0.));
#6762=DIRECTION('ref_axis',(0.,0.,-1.));
#6763=DIRECTION('center_axis',(0.,0.,1.));
#6764=DIRECTION('ref_axis',(1.,0.,0.));
#6765=DIRECTION('center_axis',(0.,-1.,0.));
#6766=DIRECTION('ref_axis',(0.,0.,-1.));
#6767=DIRECTION('center_axis',(0.,1.,0.));
#6768=DIRECTION('ref_axis',(1.,0.,0.));
#6769=DIRECTION('center_axis',(0.,-1.,0.));
#6770=DIRECTION('ref_axis',(1.,0.,0.));
#6771=DIRECTION('center_axis',(0.,-1.,0.));
#6772=DIRECTION('ref_axis',(0.,0.,-1.));
#6773=DIRECTION('center_axis',(0.,0.,1.));
#6774=DIRECTION('ref_axis',(1.,0.,0.));
#6775=DIRECTION('center_axis',(0.,-1.,0.));
#6776=DIRECTION('ref_axis',(0.,0.,-1.));
#6777=DIRECTION('center_axis',(0.,1.,0.));
#6778=DIRECTION('ref_axis',(1.,0.,0.));
#6779=DIRECTION('center_axis',(0.,-1.,0.));
#6780=DIRECTION('ref_axis',(1.,0.,0.));
#6781=DIRECTION('center_axis',(0.,-1.,0.));
#6782=DIRECTION('ref_axis',(0.,0.,-1.));
#6783=DIRECTION('center_axis',(6.12323399573676E-17,0.,1.));
#6784=DIRECTION('ref_axis',(1.,0.,0.));
#6785=DIRECTION('center_axis',(0.,-1.,0.));
#6786=DIRECTION('ref_axis',(0.,0.,-1.));
#6787=DIRECTION('center_axis',(0.,1.,0.));
#6788=DIRECTION('ref_axis',(1.,0.,0.));
#6789=DIRECTION('center_axis',(0.,-1.,0.));
#6790=DIRECTION('ref_axis',(1.,0.,0.));
#6791=DIRECTION('center_axis',(0.,-1.,0.));
#6792=DIRECTION('ref_axis',(0.,0.,-1.));
#6793=DIRECTION('center_axis',(0.,0.,1.));
#6794=DIRECTION('ref_axis',(1.,0.,0.));
#6795=DIRECTION('center_axis',(0.,-1.,0.));
#6796=DIRECTION('ref_axis',(0.,0.,-1.));
#6797=DIRECTION('center_axis',(0.,1.,0.));
#6798=DIRECTION('ref_axis',(1.,0.,0.));
#6799=DIRECTION('center_axis',(0.,1.,0.));
#6800=DIRECTION('ref_axis',(1.,0.,0.));
#6801=DIRECTION('',(0.,1.,0.));
#6802=DIRECTION('center_axis',(0.,-1.,0.));
#6803=DIRECTION('ref_axis',(1.,0.,0.));
#6804=DIRECTION('center_axis',(0.,-1.,0.));
#6805=DIRECTION('ref_axis',(1.,0.,0.));
#6806=DIRECTION('center_axis',(0.,1.,0.));
#6807=DIRECTION('ref_axis',(1.,0.,0.));
#6808=DIRECTION('center_axis',(0.,-1.,0.));
#6809=DIRECTION('ref_axis',(0.,0.,-1.));
#6810=DIRECTION('center_axis',(0.,0.,1.));
#6811=DIRECTION('ref_axis',(1.,0.,0.));
#6812=DIRECTION('center_axis',(0.,-1.,0.));
#6813=DIRECTION('ref_axis',(0.,0.,-1.));
#6814=DIRECTION('center_axis',(0.,-1.,0.));
#6815=DIRECTION('ref_axis',(-1.,0.,0.));
#6816=DIRECTION('center_axis',(0.,1.,0.));
#6817=DIRECTION('ref_axis',(1.,0.,0.));
#8874=CARTESIAN_POINT('',(0.,0.,0.));
#8875=CARTESIAN_POINT('Origin',(0.707106781186547,0.,0.707106781186548));
#8876=CARTESIAN_POINT('',(0.504455939115715,-0.04763,0.841298510752802));
#8877=CARTESIAN_POINT('',(0.841298510752802,-0.04763,0.504455939115715));
#8878=CARTESIAN_POINT('Ctrl Pts',(0.504455939115715,-0.04763,0.841298510752802));
#8879=CARTESIAN_POINT('Ctrl Pts',(0.508899795931835,-0.0740444353928835,
0.838633903678357));
#8880=CARTESIAN_POINT('Ctrl Pts',(0.517157748491652,-0.0999305678883309,
0.833661031856294));
#8881=CARTESIAN_POINT('Ctrl Pts',(0.537715343527944,-0.142345102874864,
0.820511285096538));
#8882=CARTESIAN_POINT('Ctrl Pts',(0.548874290046456,-0.159766064500479,
0.813159949759));
#8883=CARTESIAN_POINT('Ctrl Pts',(0.573915184558107,-0.190326085855194,
0.795684265985089));
#8884=CARTESIAN_POINT('Ctrl Pts',(0.587792702767295,-0.203463743702801,
0.78555112003688));
#8885=CARTESIAN_POINT('Ctrl Pts',(0.615966552324775,-0.224161999508995,
0.763642258217233));
#8886=CARTESIAN_POINT('Ctrl Pts',(0.631684198665438,-0.232861760990032,
0.750785745543687));
#8887=CARTESIAN_POINT('Ctrl Pts',(0.663382628119203,-0.244251601209411,
0.722929908501543));
#8888=CARTESIAN_POINT('Ctrl Pts',(0.679352081686668,-0.246942143572133,
0.707917883896095));
#8889=CARTESIAN_POINT('Ctrl Pts',(0.707917883896095,-0.246942143572133,
0.679352081686668));
#8890=CARTESIAN_POINT('Ctrl Pts',(0.722929908501543,-0.244251601209411,
0.663382628119203));
#8891=CARTESIAN_POINT('Ctrl Pts',(0.750785745543687,-0.232861760990032,
0.631684198665439));
#8892=CARTESIAN_POINT('Ctrl Pts',(0.763642258217232,-0.224161999508995,
0.615966552324775));
#8893=CARTESIAN_POINT('Ctrl Pts',(0.78555112003688,-0.203463743702801,0.587792702767295));
#8894=CARTESIAN_POINT('Ctrl Pts',(0.795684265985088,-0.190326085855194,
0.573915184558108));
#8895=CARTESIAN_POINT('Ctrl Pts',(0.813159949759,-0.15976606450048,0.548874290046456));
#8896=CARTESIAN_POINT('Ctrl Pts',(0.820511285096538,-0.142345102874864,
0.537715343527944));
#8897=CARTESIAN_POINT('Ctrl Pts',(0.833661031856294,-0.099930567888331,
0.517157748491653));
#8898=CARTESIAN_POINT('Ctrl Pts',(0.838633903678357,-0.0740444353928835,
0.508899795931835));
#8899=CARTESIAN_POINT('Ctrl Pts',(0.841298510752801,-0.0476299999999999,
0.504455939115715));
#8900=CARTESIAN_POINT('',(0.528110872004958,-0.04763,0.871530771444223));
#8901=CARTESIAN_POINT('Origin',(0.707106781186547,-0.04763,0.707106781186548));
#8902=CARTESIAN_POINT('',(0.871530771444223,-0.04763,0.528110872004959));
#8903=CARTESIAN_POINT('Ctrl Pts',(0.871530771444223,-0.0476300000000001,
0.528110872004958));
#8904=CARTESIAN_POINT('Ctrl Pts',(0.87014664509073,-0.0609922781173483,
0.530395067942936));
#8905=CARTESIAN_POINT('Ctrl Pts',(0.868149331745851,-0.0742967091364493,
0.533674141594226));
#8906=CARTESIAN_POINT('Ctrl Pts',(0.85981294420286,-0.115492077056649,0.54708917182331));
#8907=CARTESIAN_POINT('Ctrl Pts',(0.850993704737257,-0.141695629206859,
0.560922177770136));
#8908=CARTESIAN_POINT('Ctrl Pts',(0.830754510485543,-0.181890537957859,
0.590422647829571));
#8909=CARTESIAN_POINT('Ctrl Pts',(0.816896541396381,-0.201072148666545,
0.609616703125488));
#8910=CARTESIAN_POINT('Ctrl Pts',(0.792310597819928,-0.223955109275652,
0.641117951819998));
#8911=CARTESIAN_POINT('Ctrl Pts',(0.779109323683612,-0.232742381310829,
0.657208095763053));
#8912=CARTESIAN_POINT('Ctrl Pts',(0.750552691816206,-0.244234834628584,
0.68964083160521));
#8913=CARTESIAN_POINT('Ctrl Pts',(0.735185187071673,-0.246942143572133,
0.705971972091755));
#8914=CARTESIAN_POINT('Ctrl Pts',(0.705971972091754,-0.246942143572133,
0.735185187071673));
#8915=CARTESIAN_POINT('Ctrl Pts',(0.689640831605209,-0.244234834628584,
0.750552691816206));
#8916=CARTESIAN_POINT('Ctrl Pts',(0.657208095763052,-0.232742381310829,
0.779109323683612));
#8917=CARTESIAN_POINT('Ctrl Pts',(0.641117951819998,-0.223955109275652,
0.792310597819928));
#8918=CARTESIAN_POINT('Ctrl Pts',(0.609616703125487,-0.201072148666545,
0.816896541396382));
#8919=CARTESIAN_POINT('Ctrl Pts',(0.590422647829571,-0.181890537957858,
0.830754510485544));
#8920=CARTESIAN_POINT('Ctrl Pts',(0.560922177770135,-0.141695629206858,
0.850993704737257));
#8921=CARTESIAN_POINT('Ctrl Pts',(0.547089171823309,-0.115492077056649,
0.859812944202861));
#8922=CARTESIAN_POINT('Ctrl Pts',(0.533674141594226,-0.0742967091364491,
0.868149331745852));
#8923=CARTESIAN_POINT('Ctrl Pts',(0.530395067942936,-0.0609922781173483,
0.870146645090731));
#8924=CARTESIAN_POINT('Ctrl Pts',(0.528110872004958,-0.0476300000000001,
0.871530771444223));
#8925=CARTESIAN_POINT('Origin',(0.707106781186547,-0.04763,0.707106781186548));
#8926=CARTESIAN_POINT('Origin',(0.,-0.166705,0.));
#8927=CARTESIAN_POINT('',(0.242834539687906,-0.04763,0.989696097314));
#8928=CARTESIAN_POINT('Origin',(0.,-0.04763,0.));
#8929=CARTESIAN_POINT('',(-0.242834539687907,-0.04763,0.989696097314));
#8930=CARTESIAN_POINT('Ctrl Pts',(0.242834539687906,-0.04763,0.989696097314));
#8931=CARTESIAN_POINT('Ctrl Pts',(0.24024064412003,-0.0609922781173483,
0.990332542620729));
#8932=CARTESIAN_POINT('Ctrl Pts',(0.236509675094874,-0.0742967091364492,
0.991238884025248));
#8933=CARTESIAN_POINT('Ctrl Pts',(0.221129100087819,-0.115492077056649,
0.994830026707808));
#8934=CARTESIAN_POINT('Ctrl Pts',(0.205111543747588,-0.141695629206859,
0.998375294985966));
#8935=CARTESIAN_POINT('Ctrl Pts',(0.169940289819232,-0.181890537957859,
1.00492400591205));
#8936=CARTESIAN_POINT('Ctrl Pts',(0.1465689792446,-0.201072148666545,1.00869718865384));
#8937=CARTESIAN_POINT('Ctrl Pts',(0.106909345252087,-0.223955109275652,
1.01358704779679));
#8938=CARTESIAN_POINT('Ctrl Pts',(0.0861971848975941,-0.232742381310829,
1.0156297872271));
#8939=CARTESIAN_POINT('Ctrl Pts',(0.0430711894098822,-0.244234834628584,
1.01837060663223));
#8940=CARTESIAN_POINT('Ctrl Pts',(0.0206568624125605,-0.246942143572133,
1.019052));
#8941=CARTESIAN_POINT('Ctrl Pts',(-0.0206568624125608,-0.246942143572133,
1.019052));
#8942=CARTESIAN_POINT('Ctrl Pts',(-0.0430711894098825,-0.244234834628584,
1.01837060663223));
#8943=CARTESIAN_POINT('Ctrl Pts',(-0.0861971848975943,-0.232742381310829,
1.0156297872271));
#8944=CARTESIAN_POINT('Ctrl Pts',(-0.106909345252088,-0.223955109275652,
1.01358704779679));
#8945=CARTESIAN_POINT('Ctrl Pts',(-0.1465689792446,-0.201072148666545,1.00869718865384));
#8946=CARTESIAN_POINT('Ctrl Pts',(-0.169940289819232,-0.181890537957859,
1.00492400591205));
#8947=CARTESIAN_POINT('Ctrl Pts',(-0.205111543747588,-0.141695629206859,
0.998375294985966));
#8948=CARTESIAN_POINT('Ctrl Pts',(-0.221129100087819,-0.115492077056649,
0.994830026707808));
#8949=CARTESIAN_POINT('Ctrl Pts',(-0.236509675094875,-0.0742967091364493,
0.991238884025248));
#8950=CARTESIAN_POINT('Ctrl Pts',(-0.24024064412003,-0.0609922781173483,
0.990332542620729));
#8951=CARTESIAN_POINT('Ctrl Pts',(-0.242834539687907,-0.04763,0.989696097314));
#8952=CARTESIAN_POINT('',(-0.528110872004959,-0.04763,0.871530771444223));
#8953=CARTESIAN_POINT('Origin',(0.,-0.04763,0.));
#8954=CARTESIAN_POINT('',(-0.871530771444223,-0.04763,0.528110872004958));
#8955=CARTESIAN_POINT('Ctrl Pts',(-0.528110872004958,-0.0476300000000001,
0.871530771444223));
#8956=CARTESIAN_POINT('Ctrl Pts',(-0.530395067942936,-0.0609922781173484,
0.87014664509073));
#8957=CARTESIAN_POINT('Ctrl Pts',(-0.533674141594226,-0.0742967091364493,
0.868149331745851));
#8958=CARTESIAN_POINT('Ctrl Pts',(-0.54708917182331,-0.115492077056649,
0.85981294420286));
#8959=CARTESIAN_POINT('Ctrl Pts',(-0.560922177770136,-0.141695629206859,
0.850993704737257));
#8960=CARTESIAN_POINT('Ctrl Pts',(-0.590422647829571,-0.181890537957859,
0.830754510485543));
#8961=CARTESIAN_POINT('Ctrl Pts',(-0.609616703125488,-0.201072148666545,
0.816896541396381));
#8962=CARTESIAN_POINT('Ctrl Pts',(-0.641117951819998,-0.223955109275652,
0.792310597819928));
#8963=CARTESIAN_POINT('Ctrl Pts',(-0.657208095763053,-0.232742381310829,
0.779109323683611));
#8964=CARTESIAN_POINT('Ctrl Pts',(-0.68964083160521,-0.244234834628584,
0.750552691816205));
#8965=CARTESIAN_POINT('Ctrl Pts',(-0.705971972091755,-0.246942143572133,
0.735185187071673));
#8966=CARTESIAN_POINT('Ctrl Pts',(-0.735185187071673,-0.246942143572133,
0.705971972091754));
#8967=CARTESIAN_POINT('Ctrl Pts',(-0.750552691816206,-0.244234834628584,
0.689640831605209));
#8968=CARTESIAN_POINT('Ctrl Pts',(-0.779109323683612,-0.232742381310829,
0.657208095763052));
#8969=CARTESIAN_POINT('Ctrl Pts',(-0.792310597819928,-0.223955109275652,
0.641117951819998));
#8970=CARTESIAN_POINT('Ctrl Pts',(-0.816896541396382,-0.201072148666545,
0.609616703125487));
#8971=CARTESIAN_POINT('Ctrl Pts',(-0.830754510485544,-0.181890537957858,
0.590422647829571));
#8972=CARTESIAN_POINT('Ctrl Pts',(-0.850993704737257,-0.141695629206858,
0.560922177770135));
#8973=CARTESIAN_POINT('Ctrl Pts',(-0.859812944202861,-0.115492077056649,
0.547089171823309));
#8974=CARTESIAN_POINT('Ctrl Pts',(-0.868149331745852,-0.0742967091364491,
0.533674141594226));
#8975=CARTESIAN_POINT('Ctrl Pts',(-0.870146645090731,-0.0609922781173483,
0.530395067942936));
#8976=CARTESIAN_POINT('Ctrl Pts',(-0.871530771444223,-0.04763,0.528110872004958));
#8977=CARTESIAN_POINT('',(-0.989696097314,-0.04763,0.242834539687906));
#8978=CARTESIAN_POINT('Origin',(0.,-0.04763,0.));
#8979=CARTESIAN_POINT('',(-1.019052,-0.246942143572133,1.248489836334E-16));
#8980=CARTESIAN_POINT('Ctrl Pts',(-0.989696097314,-0.04763,0.242834539687906));
#8981=CARTESIAN_POINT('Ctrl Pts',(-0.990332542620729,-0.0609922781173483,
0.24024064412003));
#8982=CARTESIAN_POINT('Ctrl Pts',(-0.991238884025248,-0.0742967091364492,
0.236509675094874));
#8983=CARTESIAN_POINT('Ctrl Pts',(-0.994830026707808,-0.115492077056649,
0.221129100087819));
#8984=CARTESIAN_POINT('Ctrl Pts',(-0.998375294985966,-0.141695629206859,
0.205111543747588));
#8985=CARTESIAN_POINT('Ctrl Pts',(-1.00492400591205,-0.181890537957859,
0.169940289819232));
#8986=CARTESIAN_POINT('Ctrl Pts',(-1.00869718865384,-0.201072148666545,
0.1465689792446));
#8987=CARTESIAN_POINT('Ctrl Pts',(-1.01358704779679,-0.223955109275652,
0.106909345252088));
#8988=CARTESIAN_POINT('Ctrl Pts',(-1.0156297872271,-0.232742381310829,0.0861971848975944));
#8989=CARTESIAN_POINT('Ctrl Pts',(-1.01837060663223,-0.244234834628584,
0.0430711894098825));
#8990=CARTESIAN_POINT('Ctrl Pts',(-1.019052,-0.246942143572133,0.0206568624125608));
#8991=CARTESIAN_POINT('Ctrl Pts',(-1.019052,-0.246942143572133,1.2490009027033E-16));
#8992=CARTESIAN_POINT('',(-1.019052,-0.28578,1.24797876996471E-16));
#8993=CARTESIAN_POINT('',(-1.019052,-0.166705,1.24797876996471E-16));
#8994=CARTESIAN_POINT('Origin',(0.,-0.28578,0.));
#8995=CARTESIAN_POINT('',(-0.989696097314,-0.04763,-0.242834539687906));
#8996=CARTESIAN_POINT('Ctrl Pts',(-1.019052,-0.246942143572133,1.2490009027033E-16));
#8997=CARTESIAN_POINT('Ctrl Pts',(-1.019052,-0.246942143572133,-0.0206568624125605));
#8998=CARTESIAN_POINT('Ctrl Pts',(-1.01837060663223,-0.244234834628584,
-0.0430711894098822));
#8999=CARTESIAN_POINT('Ctrl Pts',(-1.0156297872271,-0.232742381310829,-0.0861971848975941));
#9000=CARTESIAN_POINT('Ctrl Pts',(-1.01358704779679,-0.223955109275652,
-0.106909345252087));
#9001=CARTESIAN_POINT('Ctrl Pts',(-1.00869718865384,-0.201072148666546,
-0.1465689792446));
#9002=CARTESIAN_POINT('Ctrl Pts',(-1.00492400591205,-0.181890537957859,
-0.169940289819232));
#9003=CARTESIAN_POINT('Ctrl Pts',(-0.998375294985966,-0.141695629206859,
-0.205111543747588));
#9004=CARTESIAN_POINT('Ctrl Pts',(-0.994830026707808,-0.11549207705665,
-0.221129100087819));
#9005=CARTESIAN_POINT('Ctrl Pts',(-0.991238884025248,-0.0742967091364495,
-0.236509675094874));
#9006=CARTESIAN_POINT('Ctrl Pts',(-0.990332542620729,-0.0609922781173484,
-0.24024064412003));
#9007=CARTESIAN_POINT('Ctrl Pts',(-0.989696097314,-0.0476300000000001,-0.242834539687907));
#9008=CARTESIAN_POINT('',(-0.871530771444223,-0.04763,-0.528110872004958));
#9009=CARTESIAN_POINT('Origin',(0.,-0.04763,0.));
#9010=CARTESIAN_POINT('',(-0.528110872004958,-0.04763,-0.871530771444223));
#9011=CARTESIAN_POINT('Ctrl Pts',(-0.871530771444223,-0.0476300000000001,
-0.528110872004958));
#9012=CARTESIAN_POINT('Ctrl Pts',(-0.87014664509073,-0.0609922781173484,
-0.530395067942936));
#9013=CARTESIAN_POINT('Ctrl Pts',(-0.868149331745851,-0.0742967091364494,
-0.533674141594226));
#9014=CARTESIAN_POINT('Ctrl Pts',(-0.85981294420286,-0.115492077056649,
-0.54708917182331));
#9015=CARTESIAN_POINT('Ctrl Pts',(-0.850993704737257,-0.141695629206859,
-0.560922177770136));
#9016=CARTESIAN_POINT('Ctrl Pts',(-0.830754510485543,-0.181890537957859,
-0.590422647829571));
#9017=CARTESIAN_POINT('Ctrl Pts',(-0.816896541396381,-0.201072148666546,
-0.609616703125488));
#9018=CARTESIAN_POINT('Ctrl Pts',(-0.792310597819928,-0.223955109275652,
-0.641117951819999));
#9019=CARTESIAN_POINT('Ctrl Pts',(-0.779109323683611,-0.232742381310829,
-0.657208095763053));
#9020=CARTESIAN_POINT('Ctrl Pts',(-0.750552691816205,-0.244234834628584,
-0.68964083160521));
#9021=CARTESIAN_POINT('Ctrl Pts',(-0.735185187071673,-0.246942143572133,
-0.705971972091755));
#9022=CARTESIAN_POINT('Ctrl Pts',(-0.705971972091754,-0.246942143572133,
-0.735185187071673));
#9023=CARTESIAN_POINT('Ctrl Pts',(-0.68964083160521,-0.244234834628584,
-0.750552691816206));
#9024=CARTESIAN_POINT('Ctrl Pts',(-0.657208095763052,-0.232742381310829,
-0.779109323683612));
#9025=CARTESIAN_POINT('Ctrl Pts',(-0.641117951819998,-0.223955109275652,
-0.792310597819928));
#9026=CARTESIAN_POINT('Ctrl Pts',(-0.609616703125488,-0.201072148666545,
-0.816896541396381));
#9027=CARTESIAN_POINT('Ctrl Pts',(-0.590422647829571,-0.181890537957859,
-0.830754510485543));
#9028=CARTESIAN_POINT('Ctrl Pts',(-0.560922177770136,-0.141695629206859,
-0.850993704737257));
#9029=CARTESIAN_POINT('Ctrl Pts',(-0.54708917182331,-0.115492077056649,
-0.85981294420286));
#9030=CARTESIAN_POINT('Ctrl Pts',(-0.533674141594226,-0.0742967091364494,
-0.868149331745852));
#9031=CARTESIAN_POINT('Ctrl Pts',(-0.530395067942936,-0.0609922781173484,
-0.870146645090731));
#9032=CARTESIAN_POINT('Ctrl Pts',(-0.528110872004958,-0.0476300000000001,
-0.871530771444223));
#9033=CARTESIAN_POINT('',(-0.242834539687906,-0.04763,-0.989696097314));
#9034=CARTESIAN_POINT('Origin',(0.,-0.04763,0.));
#9035=CARTESIAN_POINT('',(0.242834539687906,-0.04763,-0.989696097314));
#9036=CARTESIAN_POINT('Ctrl Pts',(-0.242834539687907,-0.04763,-0.989696097314));
#9037=CARTESIAN_POINT('Ctrl Pts',(-0.24024064412003,-0.0609922781173483,
-0.990332542620729));
#9038=CARTESIAN_POINT('Ctrl Pts',(-0.236509675094874,-0.0742967091364493,
-0.991238884025248));
#9039=CARTESIAN_POINT('Ctrl Pts',(-0.221129100087819,-0.115492077056649,
-0.994830026707808));
#9040=CARTESIAN_POINT('Ctrl Pts',(-0.205111543747588,-0.141695629206859,
-0.998375294985966));
#9041=CARTESIAN_POINT('Ctrl Pts',(-0.169940289819232,-0.181890537957859,
-1.00492400591205));
#9042=CARTESIAN_POINT('Ctrl Pts',(-0.1465689792446,-0.201072148666545,-1.00869718865384));
#9043=CARTESIAN_POINT('Ctrl Pts',(-0.106909345252087,-0.223955109275652,
-1.01358704779679));
#9044=CARTESIAN_POINT('Ctrl Pts',(-0.0861971848975942,-0.232742381310829,
-1.0156297872271));
#9045=CARTESIAN_POINT('Ctrl Pts',(-0.0430711894098823,-0.244234834628584,
-1.01837060663223));
#9046=CARTESIAN_POINT('Ctrl Pts',(-0.0206568624125606,-0.246942143572133,
-1.019052));
#9047=CARTESIAN_POINT('Ctrl Pts',(0.0206568624125607,-0.246942143572133,
-1.019052));
#9048=CARTESIAN_POINT('Ctrl Pts',(0.0430711894098824,-0.244234834628584,
-1.01837060663223));
#9049=CARTESIAN_POINT('Ctrl Pts',(0.0861971848975943,-0.232742381310829,
-1.0156297872271));
#9050=CARTESIAN_POINT('Ctrl Pts',(0.106909345252088,-0.223955109275652,
-1.01358704779679));
#9051=CARTESIAN_POINT('Ctrl Pts',(0.1465689792446,-0.201072148666545,-1.00869718865384));
#9052=CARTESIAN_POINT('Ctrl Pts',(0.169940289819232,-0.181890537957859,
-1.00492400591205));
#9053=CARTESIAN_POINT('Ctrl Pts',(0.205111543747588,-0.141695629206859,
-0.998375294985966));
#9054=CARTESIAN_POINT('Ctrl Pts',(0.221129100087819,-0.115492077056649,
-0.994830026707808));
#9055=CARTESIAN_POINT('Ctrl Pts',(0.236509675094874,-0.0742967091364493,
-0.991238884025248));
#9056=CARTESIAN_POINT('Ctrl Pts',(0.24024064412003,-0.0609922781173484,
-0.990332542620729));
#9057=CARTESIAN_POINT('Ctrl Pts',(0.242834539687907,-0.04763,-0.989696097314));
#9058=CARTESIAN_POINT('',(0.528110872004958,-0.04763,-0.871530771444223));
#9059=CARTESIAN_POINT('Origin',(0.,-0.04763,0.));
#9060=CARTESIAN_POINT('',(0.871530771444223,-0.04763,-0.528110872004958));
#9061=CARTESIAN_POINT('Ctrl Pts',(0.528110872004958,-0.0476300000000001,
-0.871530771444223));
#9062=CARTESIAN_POINT('Ctrl Pts',(0.530395067942936,-0.0609922781173484,
-0.870146645090731));
#9063=CARTESIAN_POINT('Ctrl Pts',(0.533674141594226,-0.0742967091364493,
-0.868149331745851));
#9064=CARTESIAN_POINT('Ctrl Pts',(0.54708917182331,-0.115492077056649,-0.85981294420286));
#9065=CARTESIAN_POINT('Ctrl Pts',(0.560922177770136,-0.141695629206859,
-0.850993704737257));
#9066=CARTESIAN_POINT('Ctrl Pts',(0.590422647829571,-0.181890537957859,
-0.830754510485543));
#9067=CARTESIAN_POINT('Ctrl Pts',(0.609616703125488,-0.201072148666545,
-0.816896541396381));
#9068=CARTESIAN_POINT('Ctrl Pts',(0.641117951819998,-0.223955109275652,
-0.792310597819928));
#9069=CARTESIAN_POINT('Ctrl Pts',(0.657208095763053,-0.232742381310829,
-0.779109323683612));
#9070=CARTESIAN_POINT('Ctrl Pts',(0.68964083160521,-0.244234834628584,-0.750552691816206));
#9071=CARTESIAN_POINT('Ctrl Pts',(0.705971972091755,-0.246942143572133,
-0.735185187071673));
#9072=CARTESIAN_POINT('Ctrl Pts',(0.735185187071673,-0.246942143572133,
-0.705971972091754));
#9073=CARTESIAN_POINT('Ctrl Pts',(0.750552691816206,-0.244234834628584,
-0.68964083160521));
#9074=CARTESIAN_POINT('Ctrl Pts',(0.779109323683612,-0.232742381310829,
-0.657208095763053));
#9075=CARTESIAN_POINT('Ctrl Pts',(0.792310597819928,-0.223955109275652,
-0.641117951819998));
#9076=CARTESIAN_POINT('Ctrl Pts',(0.816896541396381,-0.201072148666545,
-0.609616703125488));
#9077=CARTESIAN_POINT('Ctrl Pts',(0.830754510485543,-0.181890537957859,
-0.590422647829571));
#9078=CARTESIAN_POINT('Ctrl Pts',(0.850993704737257,-0.141695629206859,
-0.560922177770136));
#9079=CARTESIAN_POINT('Ctrl Pts',(0.85981294420286,-0.115492077056649,-0.54708917182331));
#9080=CARTESIAN_POINT('Ctrl Pts',(0.868149331745851,-0.0742967091364493,
-0.533674141594226));
#9081=CARTESIAN_POINT('Ctrl Pts',(0.870146645090731,-0.0609922781173484,
-0.530395067942936));
#9082=CARTESIAN_POINT('Ctrl Pts',(0.871530771444223,-0.0476300000000001,
-0.528110872004958));
#9083=CARTESIAN_POINT('',(0.989696097314,-0.04763,-0.242834539687906));
#9084=CARTESIAN_POINT('Origin',(0.,-0.04763,0.));
#9085=CARTESIAN_POINT('',(0.989696097314,-0.04763,0.242834539687906));
#9086=CARTESIAN_POINT('Ctrl Pts',(0.989696097314,-0.04763,-0.242834539687907));
#9087=CARTESIAN_POINT('Ctrl Pts',(0.990332542620729,-0.0609922781173483,
-0.24024064412003));
#9088=CARTESIAN_POINT('Ctrl Pts',(0.991238884025248,-0.0742967091364493,
-0.236509675094874));
#9089=CARTESIAN_POINT('Ctrl Pts',(0.994830026707808,-0.115492077056649,
-0.221129100087819));
#9090=CARTESIAN_POINT('Ctrl Pts',(0.998375294985966,-0.141695629206859,
-0.205111543747588));
#9091=CARTESIAN_POINT('Ctrl Pts',(1.00492400591205,-0.181890537957859,-0.169940289819232));
#9092=CARTESIAN_POINT('Ctrl Pts',(1.00869718865384,-0.201072148666545,-0.1465689792446));
#9093=CARTESIAN_POINT('Ctrl Pts',(1.01358704779679,-0.223955109275652,-0.106909345252087));
#9094=CARTESIAN_POINT('Ctrl Pts',(1.0156297872271,-0.232742381310829,-0.0861971848975942));
#9095=CARTESIAN_POINT('Ctrl Pts',(1.01837060663223,-0.244234834628584,-0.0430711894098823));
#9096=CARTESIAN_POINT('Ctrl Pts',(1.019052,-0.246942143572133,-0.0206568624125607));
#9097=CARTESIAN_POINT('Ctrl Pts',(1.019052,-0.246942143572133,0.0206568624125607));
#9098=CARTESIAN_POINT('Ctrl Pts',(1.01837060663223,-0.244234834628584,0.0430711894098823));
#9099=CARTESIAN_POINT('Ctrl Pts',(1.0156297872271,-0.232742381310829,0.0861971848975942));
#9100=CARTESIAN_POINT('Ctrl Pts',(1.01358704779679,-0.223955109275652,0.106909345252087));
#9101=CARTESIAN_POINT('Ctrl Pts',(1.00869718865384,-0.201072148666545,0.1465689792446));
#9102=CARTESIAN_POINT('Ctrl Pts',(1.00492400591205,-0.181890537957859,0.169940289819232));
#9103=CARTESIAN_POINT('Ctrl Pts',(0.998375294985966,-0.141695629206859,
0.205111543747588));
#9104=CARTESIAN_POINT('Ctrl Pts',(0.994830026707808,-0.115492077056649,
0.221129100087819));
#9105=CARTESIAN_POINT('Ctrl Pts',(0.991238884025248,-0.0742967091364492,
0.236509675094874));
#9106=CARTESIAN_POINT('Ctrl Pts',(0.990332542620729,-0.0609922781173483,
0.24024064412003));
#9107=CARTESIAN_POINT('Ctrl Pts',(0.989696097314,-0.04763,0.242834539687907));
#9108=CARTESIAN_POINT('Origin',(0.,-0.04763,0.));
#9109=CARTESIAN_POINT('Origin',(0.,-0.04763,0.));
#9110=CARTESIAN_POINT('',(0.238183666596899,-0.04763,0.951592097314));
#9111=CARTESIAN_POINT('Origin',(0.,-0.04763,0.));
#9112=CARTESIAN_POINT('Origin',(-1.94289029309402E-16,-0.04763,1.));
#9113=CARTESIAN_POINT('Origin',(-1.94289029309402E-16,0.,1.));
#9114=CARTESIAN_POINT('',(-0.2381836665969,-0.04763,0.951592097314));
#9115=CARTESIAN_POINT('Ctrl Pts',(-0.238183666596899,-0.0476299999999999,
0.951592097314));
#9116=CARTESIAN_POINT('Ctrl Pts',(-0.233157223576062,-0.0740444353928835,
0.952850216871763));
#9117=CARTESIAN_POINT('Ctrl Pts',(-0.223801617934946,-0.0999305678883309,
0.955173119738174));
#9118=CARTESIAN_POINT('Ctrl Pts',(-0.199966927975188,-0.142345102874864,
0.960411259488514));
#9119=CARTESIAN_POINT('Ctrl Pts',(-0.1868781821531,-0.159766064500479,0.963103647174702));
#9120=CARTESIAN_POINT('Ctrl Pts',(-0.15681442133453,-0.190326085855194,
0.968453058988463));
#9121=CARTESIAN_POINT('Ctrl Pts',(-0.139836317888043,-0.203463743702801,
0.971100730005489));
#9122=CARTESIAN_POINT('Ctrl Pts',(-0.104422493053067,-0.224161999508995,
0.975530745318961));
#9123=CARTESIAN_POINT('Ctrl Pts',(-0.0842175114474176,-0.232861760990032,
0.977553872336861));
#9124=CARTESIAN_POINT('Ctrl Pts',(-0.0421062857595701,-0.244251601209411,
0.980270995488453));
#9125=CARTESIAN_POINT('Ctrl Pts',(-0.0201990724523197,-0.246942143572133,
0.980948));
#9126=CARTESIAN_POINT('Ctrl Pts',(0.020199072452319,-0.246942143572133,
0.980948));
#9127=CARTESIAN_POINT('Ctrl Pts',(0.0421062857595694,-0.244251601209411,
0.980270995488454));
#9128=CARTESIAN_POINT('Ctrl Pts',(0.0842175114474169,-0.232861760990032,
0.977553872336861));
#9129=CARTESIAN_POINT('Ctrl Pts',(0.104422493053067,-0.224161999508995,
0.975530745318961));
#9130=CARTESIAN_POINT('Ctrl Pts',(0.139836317888042,-0.203463743702801,
0.971100730005489));
#9131=CARTESIAN_POINT('Ctrl Pts',(0.15681442133453,-0.190326085855194,0.968453058988463));
#9132=CARTESIAN_POINT('Ctrl Pts',(0.1868781821531,-0.15976606450048,0.963103647174702));
#9133=CARTESIAN_POINT('Ctrl Pts',(0.199966927975188,-0.142345102874864,
0.960411259488514));
#9134=CARTESIAN_POINT('Ctrl Pts',(0.223801617934945,-0.0999305678883309,
0.955173119738174));
#9135=CARTESIAN_POINT('Ctrl Pts',(0.233157223576061,-0.0740444353928835,
0.952850216871763));
#9136=CARTESIAN_POINT('Ctrl Pts',(0.238183666596899,-0.0476299999999999,
0.951592097314));
#9137=CARTESIAN_POINT('Origin',(-1.94289029309402E-16,-0.04763,1.));
#9138=CARTESIAN_POINT('Origin',(0.,-0.04763,0.));
#9139=CARTESIAN_POINT('',(-0.504455939115715,-0.04763,0.841298510752802));
#9140=CARTESIAN_POINT('Origin',(0.,-0.04763,0.));
#9141=CARTESIAN_POINT('Origin',(-0.707106781186548,-0.04763,0.707106781186547));
#9142=CARTESIAN_POINT('Origin',(-0.707106781186548,0.,0.707106781186547));
#9143=CARTESIAN_POINT('',(-0.841298510752802,-0.04763,0.504455939115715));
#9144=CARTESIAN_POINT('Ctrl Pts',(-0.841298510752802,-0.04763,0.504455939115715));
#9145=CARTESIAN_POINT('Ctrl Pts',(-0.838633903678357,-0.0740444353928835,
0.508899795931835));
#9146=CARTESIAN_POINT('Ctrl Pts',(-0.833661031856294,-0.0999305678883309,
0.517157748491652));
#9147=CARTESIAN_POINT('Ctrl Pts',(-0.820511285096538,-0.142345102874864,
0.537715343527944));
#9148=CARTESIAN_POINT('Ctrl Pts',(-0.813159949759,-0.159766064500479,0.548874290046456));
#9149=CARTESIAN_POINT('Ctrl Pts',(-0.795684265985089,-0.190326085855194,
0.573915184558107));
#9150=CARTESIAN_POINT('Ctrl Pts',(-0.78555112003688,-0.203463743702801,
0.587792702767295));
#9151=CARTESIAN_POINT('Ctrl Pts',(-0.763642258217233,-0.224161999508995,
0.615966552324775));
#9152=CARTESIAN_POINT('Ctrl Pts',(-0.750785745543687,-0.232861760990032,
0.631684198665438));
#9153=CARTESIAN_POINT('Ctrl Pts',(-0.722929908501543,-0.244251601209411,
0.663382628119203));
#9154=CARTESIAN_POINT('Ctrl Pts',(-0.707917883896095,-0.246942143572133,
0.679352081686668));
#9155=CARTESIAN_POINT('Ctrl Pts',(-0.679352081686668,-0.246942143572133,
0.707917883896095));
#9156=CARTESIAN_POINT('Ctrl Pts',(-0.663382628119203,-0.244251601209411,
0.722929908501544));
#9157=CARTESIAN_POINT('Ctrl Pts',(-0.631684198665438,-0.232861760990031,
0.750785745543687));
#9158=CARTESIAN_POINT('Ctrl Pts',(-0.615966552324775,-0.224161999508995,
0.763642258217233));
#9159=CARTESIAN_POINT('Ctrl Pts',(-0.587792702767295,-0.203463743702801,
0.78555112003688));
#9160=CARTESIAN_POINT('Ctrl Pts',(-0.573915184558107,-0.190326085855194,
0.795684265985088));
#9161=CARTESIAN_POINT('Ctrl Pts',(-0.548874290046456,-0.159766064500479,
0.813159949759));
#9162=CARTESIAN_POINT('Ctrl Pts',(-0.537715343527944,-0.142345102874864,
0.820511285096538));
#9163=CARTESIAN_POINT('Ctrl Pts',(-0.517157748491652,-0.0999305678883309,
0.833661031856294));
#9164=CARTESIAN_POINT('Ctrl Pts',(-0.508899795931835,-0.0740444353928835,
0.838633903678357));
#9165=CARTESIAN_POINT('Ctrl Pts',(-0.504455939115716,-0.04763,0.841298510752801));
#9166=CARTESIAN_POINT('Origin',(-0.707106781186548,-0.04763,0.707106781186547));
#9167=CARTESIAN_POINT('Origin',(0.,-0.04763,0.));
#9168=CARTESIAN_POINT('',(-0.951592097314,-0.04763,0.238183666596899));
#9169=CARTESIAN_POINT('Origin',(0.,-0.04763,0.));
#9170=CARTESIAN_POINT('Origin',(-1.,-0.04763,-1.11022302462516E-16));
#9171=CARTESIAN_POINT('Origin',(-1.,0.,-1.11022302462516E-16));
#9172=CARTESIAN_POINT('',(-0.951592097314,-0.04763,-0.2381836665969));
#9173=CARTESIAN_POINT('',(-0.980948,-0.246942143572133,1.08514323328844E-18));
#9174=CARTESIAN_POINT('Ctrl Pts',(-0.951592097314,-0.04763,-0.238183666596899));
#9175=CARTESIAN_POINT('Ctrl Pts',(-0.952850216871763,-0.0740444353928835,
-0.233157223576062));
#9176=CARTESIAN_POINT('Ctrl Pts',(-0.955173119738174,-0.0999305678883309,
-0.223801617934946));
#9177=CARTESIAN_POINT('Ctrl Pts',(-0.960411259488514,-0.142345102874864,
-0.199966927975188));
#9178=CARTESIAN_POINT('Ctrl Pts',(-0.963103647174702,-0.159766064500479,
-0.1868781821531));
#9179=CARTESIAN_POINT('Ctrl Pts',(-0.968453058988463,-0.190326085855194,
-0.15681442133453));
#9180=CARTESIAN_POINT('Ctrl Pts',(-0.971100730005489,-0.203463743702801,
-0.139836317888043));
#9181=CARTESIAN_POINT('Ctrl Pts',(-0.975530745318961,-0.224161999508995,
-0.104422493053067));
#9182=CARTESIAN_POINT('Ctrl Pts',(-0.977553872336861,-0.232861760990032,
-0.0842175114474175));
#9183=CARTESIAN_POINT('Ctrl Pts',(-0.980270995488453,-0.244251601209411,
-0.0421062857595699));
#9184=CARTESIAN_POINT('Ctrl Pts',(-0.980948,-0.246942143572133,-0.0201990724523195));
#9185=CARTESIAN_POINT('Ctrl Pts',(-0.980948,-0.246942143572133,-1.17961196366423E-16));
#9186=CARTESIAN_POINT('Origin',(-1.,-0.04763,-1.11022302462516E-16));
#9187=CARTESIAN_POINT('Ctrl Pts',(-0.980948,-0.246942143572133,-1.17961196366423E-16));
#9188=CARTESIAN_POINT('Ctrl Pts',(-0.980948,-0.246942143572133,0.0201990724523192));
#9189=CARTESIAN_POINT('Ctrl Pts',(-0.980270995488453,-0.244251601209411,
0.0421062857595695));
#9190=CARTESIAN_POINT('Ctrl Pts',(-0.977553872336861,-0.232861760990032,
0.0842175114474169));
#9191=CARTESIAN_POINT('Ctrl Pts',(-0.975530745318961,-0.224161999508995,
0.104422493053066));
#9192=CARTESIAN_POINT('Ctrl Pts',(-0.971100730005489,-0.203463743702801,
0.139836317888042));
#9193=CARTESIAN_POINT('Ctrl Pts',(-0.968453058988463,-0.190326085855194,
0.15681442133453));
#9194=CARTESIAN_POINT('Ctrl Pts',(-0.963103647174702,-0.15976606450048,
0.1868781821531));
#9195=CARTESIAN_POINT('Ctrl Pts',(-0.960411259488514,-0.142345102874864,
0.199966927975188));
#9196=CARTESIAN_POINT('Ctrl Pts',(-0.955173119738174,-0.099930567888331,
0.223801617934945));
#9197=CARTESIAN_POINT('Ctrl Pts',(-0.952850216871763,-0.0740444353928835,
0.233157223576061));
#9198=CARTESIAN_POINT('Ctrl Pts',(-0.951592097314,-0.04763,0.238183666596899));
#9199=CARTESIAN_POINT('Origin',(0.,-0.04763,0.));
#9200=CARTESIAN_POINT('',(-0.841298510752802,-0.04763,-0.504455939115715));
#9201=CARTESIAN_POINT('Origin',(0.,-0.04763,0.));
#9202=CARTESIAN_POINT('Origin',(-0.707106781186547,-0.04763,-0.707106781186548));
#9203=CARTESIAN_POINT('Origin',(-0.707106781186547,0.,-0.707106781186548));
#9204=CARTESIAN_POINT('',(-0.504455939115715,-0.04763,-0.841298510752802));
#9205=CARTESIAN_POINT('Ctrl Pts',(-0.504455939115715,-0.04763,-0.841298510752802));
#9206=CARTESIAN_POINT('Ctrl Pts',(-0.508899795931835,-0.0740444353928835,
-0.838633903678357));
#9207=CARTESIAN_POINT('Ctrl Pts',(-0.517157748491652,-0.0999305678883309,
-0.833661031856294));
#9208=CARTESIAN_POINT('Ctrl Pts',(-0.537715343527944,-0.142345102874864,
-0.820511285096538));
#9209=CARTESIAN_POINT('Ctrl Pts',(-0.548874290046456,-0.159766064500479,
-0.813159949759));
#9210=CARTESIAN_POINT('Ctrl Pts',(-0.573915184558107,-0.190326085855194,
-0.795684265985089));
#9211=CARTESIAN_POINT('Ctrl Pts',(-0.587792702767295,-0.203463743702801,
-0.78555112003688));
#9212=CARTESIAN_POINT('Ctrl Pts',(-0.615966552324775,-0.224161999508995,
-0.763642258217233));
#9213=CARTESIAN_POINT('Ctrl Pts',(-0.631684198665438,-0.232861760990032,
-0.750785745543687));
#9214=CARTESIAN_POINT('Ctrl Pts',(-0.663382628119203,-0.244251601209411,
-0.722929908501543));
#9215=CARTESIAN_POINT('Ctrl Pts',(-0.679352081686668,-0.246942143572133,
-0.707917883896095));
#9216=CARTESIAN_POINT('Ctrl Pts',(-0.707917883896095,-0.246942143572133,
-0.679352081686668));
#9217=CARTESIAN_POINT('Ctrl Pts',(-0.722929908501543,-0.244251601209411,
-0.663382628119203));
#9218=CARTESIAN_POINT('Ctrl Pts',(-0.750785745543687,-0.232861760990032,
-0.631684198665439));
#9219=CARTESIAN_POINT('Ctrl Pts',(-0.763642258217232,-0.224161999508995,
-0.615966552324775));
#9220=CARTESIAN_POINT('Ctrl Pts',(-0.78555112003688,-0.203463743702801,
-0.587792702767295));
#9221=CARTESIAN_POINT('Ctrl Pts',(-0.795684265985088,-0.190326085855194,
-0.573915184558107));
#9222=CARTESIAN_POINT('Ctrl Pts',(-0.813159949759,-0.15976606450048,-0.548874290046456));
#9223=CARTESIAN_POINT('Ctrl Pts',(-0.820511285096538,-0.142345102874864,
-0.537715343527944));
#9224=CARTESIAN_POINT('Ctrl Pts',(-0.833661031856294,-0.0999305678883311,
-0.517157748491652));
#9225=CARTESIAN_POINT('Ctrl Pts',(-0.838633903678357,-0.0740444353928836,
-0.508899795931835));
#9226=CARTESIAN_POINT('Ctrl Pts',(-0.841298510752801,-0.04763,-0.504455939115715));
#9227=CARTESIAN_POINT('Origin',(-0.707106781186547,-0.04763,-0.707106781186548));
#9228=CARTESIAN_POINT('Origin',(0.,-0.04763,0.));
#9229=CARTESIAN_POINT('',(-0.238183666596899,-0.04763,-0.951592097314));
#9230=CARTESIAN_POINT('Origin',(0.,-0.04763,0.));
#9231=CARTESIAN_POINT('Origin',(5.55111512312578E-17,-0.04763,-1.));
#9232=CARTESIAN_POINT('Origin',(5.55111512312578E-17,0.,-1.));
#9233=CARTESIAN_POINT('',(0.238183666596899,-0.04763,-0.951592097314));
#9234=CARTESIAN_POINT('Ctrl Pts',(0.238183666596899,-0.04763,-0.951592097314));
#9235=CARTESIAN_POINT('Ctrl Pts',(0.233157223576062,-0.0740444353928835,
-0.952850216871763));
#9236=CARTESIAN_POINT('Ctrl Pts',(0.223801617934946,-0.099930567888331,
-0.955173119738174));
#9237=CARTESIAN_POINT('Ctrl Pts',(0.199966927975188,-0.142345102874864,
-0.960411259488514));
#9238=CARTESIAN_POINT('Ctrl Pts',(0.1868781821531,-0.15976606450048,-0.963103647174702));
#9239=CARTESIAN_POINT('Ctrl Pts',(0.15681442133453,-0.190326085855194,-0.968453058988463));
#9240=CARTESIAN_POINT('Ctrl Pts',(0.139836317888042,-0.203463743702801,
-0.971100730005489));
#9241=CARTESIAN_POINT('Ctrl Pts',(0.104422493053067,-0.224161999508995,
-0.975530745318961));
#9242=CARTESIAN_POINT('Ctrl Pts',(0.0842175114474173,-0.232861760990032,
-0.977553872336861));
#9243=CARTESIAN_POINT('Ctrl Pts',(0.0421062857595698,-0.244251601209411,
-0.980270995488453));
#9244=CARTESIAN_POINT('Ctrl Pts',(0.0201990724523194,-0.246942143572133,
-0.980948));
#9245=CARTESIAN_POINT('Ctrl Pts',(-0.0201990724523193,-0.246942143572133,
-0.980948));
#9246=CARTESIAN_POINT('Ctrl Pts',(-0.0421062857595697,-0.244251601209411,
-0.980270995488453));
#9247=CARTESIAN_POINT('Ctrl Pts',(-0.0842175114474171,-0.232861760990032,
-0.977553872336861));
#9248=CARTESIAN_POINT('Ctrl Pts',(-0.104422493053067,-0.224161999508995,
-0.975530745318961));
#9249=CARTESIAN_POINT('Ctrl Pts',(-0.139836317888042,-0.203463743702801,
-0.971100730005489));
#9250=CARTESIAN_POINT('Ctrl Pts',(-0.15681442133453,-0.190326085855194,
-0.968453058988463));
#9251=CARTESIAN_POINT('Ctrl Pts',(-0.1868781821531,-0.15976606450048,-0.963103647174702));
#9252=CARTESIAN_POINT('Ctrl Pts',(-0.199966927975188,-0.142345102874864,
-0.960411259488514));
#9253=CARTESIAN_POINT('Ctrl Pts',(-0.223801617934945,-0.099930567888331,
-0.955173119738174));
#9254=CARTESIAN_POINT('Ctrl Pts',(-0.233157223576062,-0.0740444353928835,
-0.952850216871763));
#9255=CARTESIAN_POINT('Ctrl Pts',(-0.238183666596899,-0.0476299999999999,
-0.951592097314));
#9256=CARTESIAN_POINT('Origin',(5.55111512312578E-17,-0.04763,-1.));
#9257=CARTESIAN_POINT('Origin',(0.,-0.04763,0.));
#9258=CARTESIAN_POINT('',(0.504455939115715,-0.04763,-0.841298510752802));
#9259=CARTESIAN_POINT('Origin',(0.,-0.04763,0.));
#9260=CARTESIAN_POINT('Origin',(0.707106781186548,-0.04763,-0.707106781186547));
#9261=CARTESIAN_POINT('Origin',(0.707106781186548,0.,-0.707106781186547));
#9262=CARTESIAN_POINT('',(0.841298510752802,-0.04763,-0.504455939115715));
#9263=CARTESIAN_POINT('Ctrl Pts',(0.841298510752802,-0.04763,-0.504455939115715));
#9264=CARTESIAN_POINT('Ctrl Pts',(0.838633903678357,-0.0740444353928835,
-0.508899795931835));
#9265=CARTESIAN_POINT('Ctrl Pts',(0.833661031856294,-0.0999305678883309,
-0.517157748491652));
#9266=CARTESIAN_POINT('Ctrl Pts',(0.820511285096538,-0.142345102874864,
-0.537715343527944));
#9267=CARTESIAN_POINT('Ctrl Pts',(0.813159949759,-0.159766064500479,-0.548874290046456));
#9268=CARTESIAN_POINT('Ctrl Pts',(0.795684265985088,-0.190326085855194,
-0.573915184558107));
#9269=CARTESIAN_POINT('Ctrl Pts',(0.78555112003688,-0.203463743702801,-0.587792702767295));
#9270=CARTESIAN_POINT('Ctrl Pts',(0.763642258217233,-0.224161999508995,
-0.615966552324775));
#9271=CARTESIAN_POINT('Ctrl Pts',(0.750785745543687,-0.232861760990032,
-0.631684198665438));
#9272=CARTESIAN_POINT('Ctrl Pts',(0.722929908501543,-0.244251601209411,
-0.663382628119203));
#9273=CARTESIAN_POINT('Ctrl Pts',(0.707917883896095,-0.246942143572133,
-0.679352081686668));
#9274=CARTESIAN_POINT('Ctrl Pts',(0.679352081686668,-0.246942143572133,
-0.707917883896095));
#9275=CARTESIAN_POINT('Ctrl Pts',(0.663382628119203,-0.244251601209411,
-0.722929908501543));
#9276=CARTESIAN_POINT('Ctrl Pts',(0.631684198665438,-0.232861760990032,
-0.750785745543687));
#9277=CARTESIAN_POINT('Ctrl Pts',(0.615966552324775,-0.224161999508995,
-0.763642258217232));
#9278=CARTESIAN_POINT('Ctrl Pts',(0.587792702767295,-0.203463743702801,
-0.78555112003688));
#9279=CARTESIAN_POINT('Ctrl Pts',(0.573915184558107,-0.190326085855194,
-0.795684265985088));
#9280=CARTESIAN_POINT('Ctrl Pts',(0.548874290046456,-0.159766064500479,
-0.813159949759));
#9281=CARTESIAN_POINT('Ctrl Pts',(0.537715343527944,-0.142345102874864,
-0.820511285096538));
#9282=CARTESIAN_POINT('Ctrl Pts',(0.517157748491652,-0.099930567888331,
-0.833661031856294));
#9283=CARTESIAN_POINT('Ctrl Pts',(0.508899795931835,-0.0740444353928835,
-0.838633903678357));
#9284=CARTESIAN_POINT('Ctrl Pts',(0.504455939115715,-0.04763,-0.841298510752801));
#9285=CARTESIAN_POINT('Origin',(0.707106781186548,-0.04763,-0.707106781186547));
#9286=CARTESIAN_POINT('Origin',(0.,-0.166705,0.));
#9287=CARTESIAN_POINT('',(-0.980948,-0.28578,1.20131482833E-16));
#9288=CARTESIAN_POINT('Origin',(0.,-0.28578,0.));
#9289=CARTESIAN_POINT('',(-0.980948,-0.166705,1.20131482833E-16));
#9290=CARTESIAN_POINT('',(0.951592097314,-0.04763,0.238183666596899));
#9291=CARTESIAN_POINT('Origin',(0.,-0.04763,0.));
#9292=CARTESIAN_POINT('',(0.951592097314,-0.04763,-0.238183666596899));
#9293=CARTESIAN_POINT('Ctrl Pts',(0.951592097314,-0.04763,0.238183666596899));
#9294=CARTESIAN_POINT('Ctrl Pts',(0.952850216871763,-0.0740444353928835,
0.233157223576062));
#9295=CARTESIAN_POINT('Ctrl Pts',(0.955173119738174,-0.099930567888331,
0.223801617934945));
#9296=CARTESIAN_POINT('Ctrl Pts',(0.960411259488514,-0.142345102874864,
0.199966927975188));
#9297=CARTESIAN_POINT('Ctrl Pts',(0.963103647174702,-0.15976606450048,0.1868781821531));
#9298=CARTESIAN_POINT('Ctrl Pts',(0.968453058988463,-0.190326085855194,
0.15681442133453));
#9299=CARTESIAN_POINT('Ctrl Pts',(0.971100730005489,-0.203463743702801,
0.139836317888042));
#9300=CARTESIAN_POINT('Ctrl Pts',(0.975530745318961,-0.224161999508995,
0.104422493053067));
#9301=CARTESIAN_POINT('Ctrl Pts',(0.977553872336861,-0.232861760990032,
0.0842175114474172));
#9302=CARTESIAN_POINT('Ctrl Pts',(0.980270995488453,-0.244251601209411,
0.0421062857595697));
#9303=CARTESIAN_POINT('Ctrl Pts',(0.980948,-0.246942143572133,0.0201990724523194));
#9304=CARTESIAN_POINT('Ctrl Pts',(0.980948,-0.246942143572133,-0.0201990724523194));
#9305=CARTESIAN_POINT('Ctrl Pts',(0.980270995488453,-0.244251601209411,
-0.0421062857595697));
#9306=CARTESIAN_POINT('Ctrl Pts',(0.977553872336861,-0.232861760990032,
-0.0842175114474172));
#9307=CARTESIAN_POINT('Ctrl Pts',(0.975530745318961,-0.224161999508995,
-0.104422493053067));
#9308=CARTESIAN_POINT('Ctrl Pts',(0.971100730005489,-0.203463743702801,
-0.139836317888042));
#9309=CARTESIAN_POINT('Ctrl Pts',(0.968453058988463,-0.190326085855194,
-0.15681442133453));
#9310=CARTESIAN_POINT('Ctrl Pts',(0.963103647174702,-0.15976606450048,-0.1868781821531));
#9311=CARTESIAN_POINT('Ctrl Pts',(0.960411259488514,-0.142345102874864,
-0.199966927975188));
#9312=CARTESIAN_POINT('Ctrl Pts',(0.955173119738174,-0.099930567888331,
-0.223801617934945));
#9313=CARTESIAN_POINT('Ctrl Pts',(0.952850216871763,-0.0740444353928835,
-0.233157223576062));
#9314=CARTESIAN_POINT('Ctrl Pts',(0.951592097314,-0.0476299999999999,-0.238183666596899));
#9315=CARTESIAN_POINT('Origin',(0.,-0.04763,0.));
#9316=CARTESIAN_POINT('Origin',(0.,-0.04763,0.));
#9317=CARTESIAN_POINT('Origin',(1.,-0.04763,0.));
#9318=CARTESIAN_POINT('Origin',(1.,0.,0.));
#9319=CARTESIAN_POINT('Origin',(1.,-0.04763,0.));
#9320=CARTESIAN_POINT('Origin',(0.,-0.28578,0.));
#9321=CARTESIAN_POINT('Origin',(0.,-0.04763,0.));
#9767=UNCERTAINTY_MEASURE_WITH_UNIT(LENGTH_MEASURE(0.001),#9814,
'DISTANCE_ACCURACY_VALUE',
'Maximum model space distance between geometric entities at asserted c
onnectivities');
#9777=UNCERTAINTY_MEASURE_WITH_UNIT(LENGTH_MEASURE(0.001),#9814,
'DISTANCE_ACCURACY_VALUE',
'Maximum model space distance between geometric entities at asserted c
onnectivities');
#9803=(
GEOMETRIC_REPRESENTATION_CONTEXT(3)
GLOBAL_UNCERTAINTY_ASSIGNED_CONTEXT((#9767))
GLOBAL_UNIT_ASSIGNED_CONTEXT((#9814,#9816,#9817))
REPRESENTATION_CONTEXT('','3D')
);
#9813=(
GEOMETRIC_REPRESENTATION_CONTEXT(3)
GLOBAL_UNCERTAINTY_ASSIGNED_CONTEXT((#9777))
GLOBAL_UNIT_ASSIGNED_CONTEXT((#9814,#9816,#9817))
REPRESENTATION_CONTEXT('','3D')
);
#9814=(
LENGTH_UNIT()
NAMED_UNIT(*)
SI_UNIT(.CENTI.,.METRE.)
);
#9816=(
NAMED_UNIT(*)
PLANE_ANGLE_UNIT()
SI_UNIT($,.RADIAN.)
);
#9817=(
NAMED_UNIT(*)
SI_UNIT($,.STERADIAN.)
SOLID_ANGLE_UNIT()
);
#9843=SHAPE_DEFINITION_REPRESENTATION(#9878,#9960);
#9878=PRODUCT_DEFINITION_SHAPE('',$,#9996);
#9960=SHAPE_REPRESENTATION('',(#5500),#9803);
#9970=PRODUCT_DEFINITION_CONTEXT('part definition',#10077,'design');
#9996=PRODUCT_DEFINITION('Cage','Cage',#10031,#9970);
#10031=PRODUCT_DEFINITION_FORMATION('',$,#10104);
#10077=APPLICATION_CONTEXT(
'Core Data for Automotive Mechanical Design Process');
#10078=PRODUCT_CONTEXT('part definition',#10077,'mechanical');
#10104=PRODUCT('Cage','Cage','Cage',(#10078));
#10177=COLOUR_RGB('Grey',0.48,0.52,0.57);
#10178=FILL_AREA_STYLE_COLOUR('',#10177);
#10179=FILL_AREA_STYLE('',(#10178));
#10180=SURFACE_STYLE_FILL_AREA(#10179);
#10181=SURFACE_SIDE_STYLE('',(#10180));
#10182=SURFACE_STYLE_USAGE(.BOTH.,#10181);
#10183=PRESENTATION_STYLE_ASSIGNMENT((#10182));
ENDSEC;
END-ISO-10303-21;
